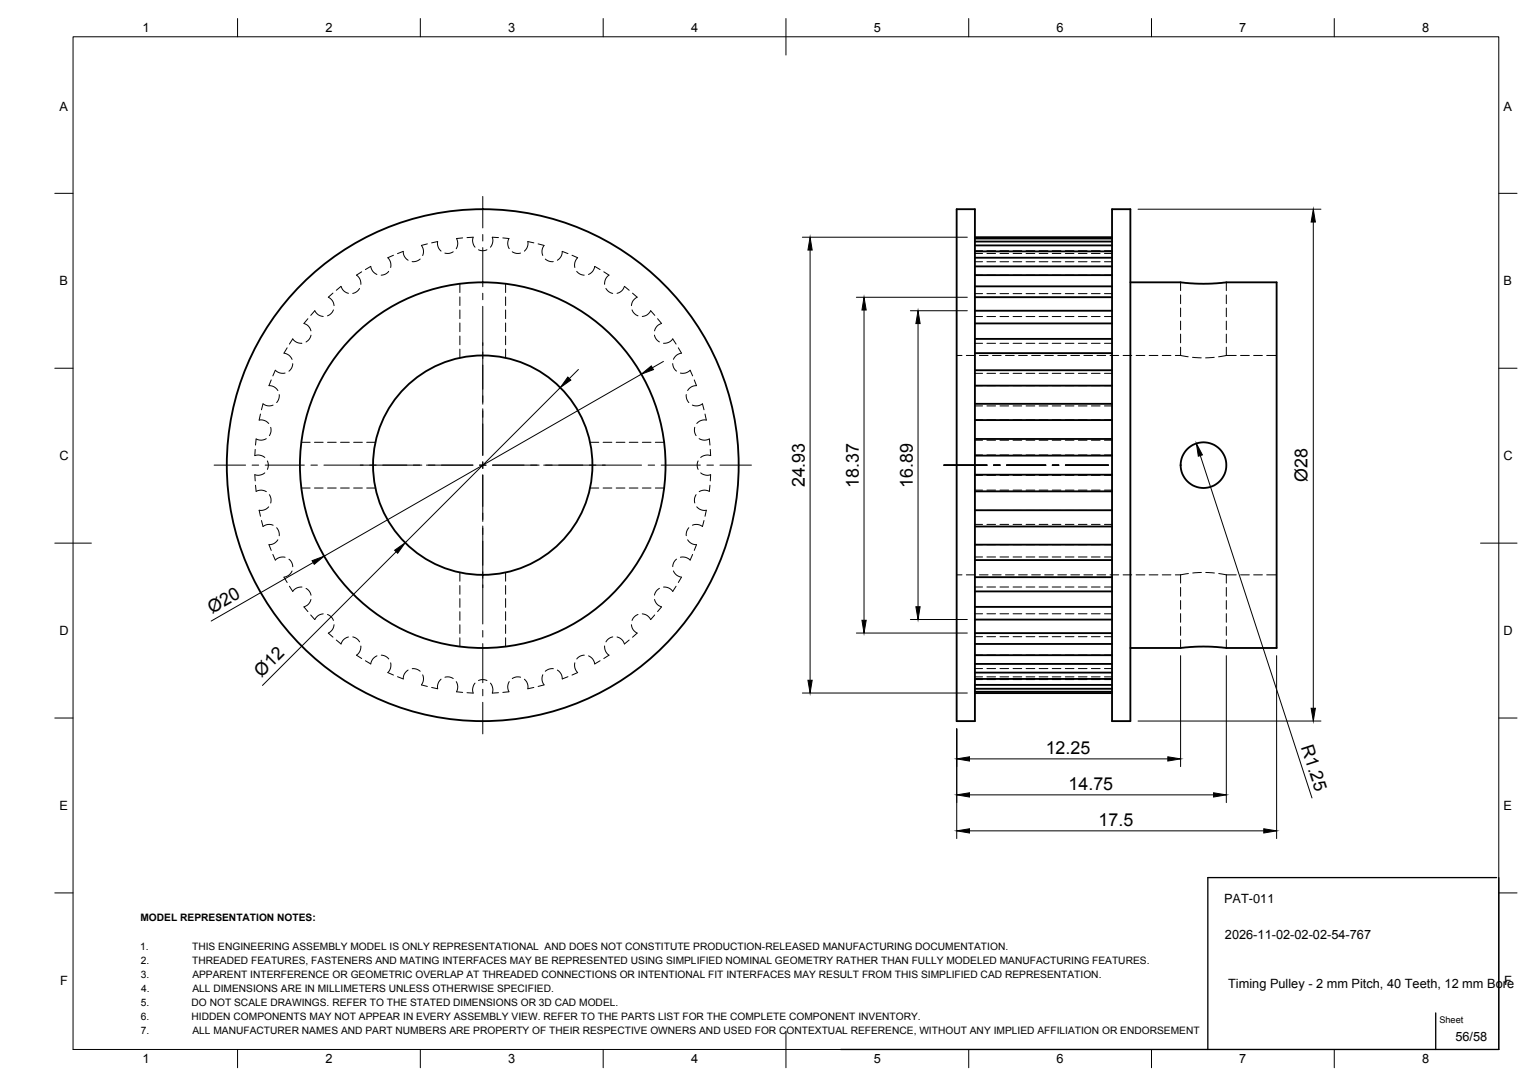
ISO-10303-21;
HEADER;
/* Generated by software containing ST-Developer
 * from STEP Tools, Inc. (www.steptools.com) 
 */

FILE_DESCRIPTION(
/* description */ ('Belt tension measurement rig'),
/* implementation_level */ '2;1');

FILE_NAME(
/* name */ 'Timing Pulley - 2 mm Pitch, 40 Teeth, 12 mm Bore.step',
/* time_stamp */ '2026-10-28T03:24:44-07:00',
/* author */ (''),
/* organization */ (''),
/* preprocessor_version */ 'ST-DEVELOPER v20.2',
/* originating_system */ 'Autodesk Translation Framework v15.17.0.0',
/* authorisation */ '');

FILE_SCHEMA (('AUTOMOTIVE_DESIGN { 1 0 10303 214 3 1 1 }'));
ENDSEC;

DATA;
#10=MECHANICAL_DESIGN_GEOMETRIC_PRESENTATION_REPRESENTATION('',(#757),#23587);
#553=B_SPLINE_CURVE_WITH_KNOTS('',3,(#22249,#22250,#22251,#22252,#22253,
#22254,#22255,#22256,#22257,#22258),.UNSPECIFIED.,.F.,.F.,(4,2,2,2,4),(0.565665723963061,
0.61280433739166,0.659942950820258,0.70708195805217,0.754220965284082),
 .UNSPECIFIED.);
#554=B_SPLINE_CURVE_WITH_KNOTS('',3,(#22260,#22261,#22262,#22263,#22264,
#22265,#22266,#22267,#22268,#22269,#22270,#22271,#22272,#22273,#22274,#22275,
#22276,#22277),.UNSPECIFIED.,.F.,.F.,(4,2,2,2,2,2,2,2,4),(0.18855524132102,
0.235693854749619,0.282832468178217,0.329971475410129,0.377110482642041,
0.424249489873953,0.471388497105864,0.518527110534463,0.565665723963061),
 .UNSPECIFIED.);
#555=B_SPLINE_CURVE_WITH_KNOTS('',3,(#22278,#22279,#22280,#22281,#22282,
#22283,#22284,#22285,#22286,#22287),.UNSPECIFIED.,.F.,.F.,(4,2,2,2,4),(0.754220965284082,
0.801359972515993,0.848498979747905,0.895637593176504,0.942776206605102),
 .UNSPECIFIED.);
#556=B_SPLINE_CURVE_WITH_KNOTS('',3,(#22291,#22292,#22293,#22294,#22295,
#22296,#22297,#22298,#22299,#22300),.UNSPECIFIED.,.F.,.F.,(4,2,2,2,4),(0.188940047579712,
0.236173496177583,0.283406944775455,0.330643519967439,0.377880095159423),
 .UNSPECIFIED.);
#557=B_SPLINE_CURVE_WITH_KNOTS('',3,(#22302,#22303,#22304,#22305,#22306,
#22307,#22308,#22309,#22310,#22311),.UNSPECIFIED.,.F.,.F.,(4,2,2,2,4),(0.,
0.0472365751919841,0.0944731503839682,0.14170659898184,0.188940047579712),
 .UNSPECIFIED.);
#558=B_SPLINE_CURVE_WITH_KNOTS('',3,(#22313,#22314,#22315,#22316,#22317,
#22318,#22319,#22320,#22321,#22322),.UNSPECIFIED.,.F.,.F.,(4,2,2,2,4),(0.566820142739135,
0.614053591337007,0.661287039934879,0.708523615126863,0.755760190318847),
 .UNSPECIFIED.);
#559=B_SPLINE_CURVE_WITH_KNOTS('',3,(#22323,#22324,#22325,#22326,#22327,
#22328,#22329,#22330,#22331,#22332),.UNSPECIFIED.,.F.,.F.,(4,2,2,2,4),(0.377880095159423,
0.425116670351408,0.472353245543392,0.519586694141263,0.566820142739135),
 .UNSPECIFIED.);
#560=B_SPLINE_CURVE_WITH_KNOTS('',3,(#22336,#22337,#22338,#22339,#22340,
#22341,#22342,#22343,#22344,#22345,#22346,#22347,#22348,#22349,#22350,#22351,
#22352,#22353),.UNSPECIFIED.,.F.,.F.,(4,2,2,2,2,2,2,2,4),(0.,0.0472365751919841,
0.0944731503839683,0.14170659898184,0.188940047579712,0.236173496177583,
0.283406944775455,0.330643519967439,0.377880095159423),.UNSPECIFIED.);
#561=B_SPLINE_CURVE_WITH_KNOTS('',3,(#22354,#22355,#22356,#22357,#22358,
#22359,#22360,#22361,#22362,#22363,#22364,#22365,#22366,#22367,#22368,#22369,
#22370,#22371),.UNSPECIFIED.,.F.,.F.,(4,2,2,2,2,2,2,2,4),(0.377880095159423,
0.425116670351408,0.472353245543392,0.519586694141263,0.566820142739135,
0.614053591337007,0.661287039934879,0.708523615126863,0.755760190318847),
 .UNSPECIFIED.);
#562=B_SPLINE_CURVE_WITH_KNOTS('',3,(#22375,#22376,#22377,#22378,#22379,
#22380,#22381,#22382,#22383,#22384),.UNSPECIFIED.,.F.,.F.,(4,2,2,2,4),(0.565665723963061,
0.61280433739166,0.659942950820258,0.70708195805217,0.754220965284082),
 .UNSPECIFIED.);
#563=B_SPLINE_CURVE_WITH_KNOTS('',3,(#22386,#22387,#22388,#22389,#22390,
#22391,#22392,#22393,#22394,#22395,#22396,#22397,#22398,#22399,#22400,#22401,
#22402,#22403),.UNSPECIFIED.,.F.,.F.,(4,2,2,2,2,2,2,2,4),(0.18855524132102,
0.235693854749619,0.282832468178217,0.329971475410129,0.377110482642041,
0.424249489873953,0.471388497105864,0.518527110534463,0.565665723963061),
 .UNSPECIFIED.);
#564=B_SPLINE_CURVE_WITH_KNOTS('',3,(#22404,#22405,#22406,#22407,#22408,
#22409,#22410,#22411,#22412,#22413),.UNSPECIFIED.,.F.,.F.,(4,2,2,2,4),(0.754220965284082,
0.801359972515993,0.848498979747905,0.895637593176504,0.942776206605102),
 .UNSPECIFIED.);
#565=B_SPLINE_CURVE_WITH_KNOTS('',3,(#22423,#22424,#22425,#22426,#22427,
#22428,#22429,#22430,#22431,#22432,#22433,#22434,#22435,#22436,#22437,#22438,
#22439,#22440),.UNSPECIFIED.,.F.,.F.,(4,2,2,2,2,2,2,2,4),(0.18855524132102,
0.235693854749619,0.282832468178217,0.329971475410129,0.377110482642041,
0.424249489873953,0.471388497105864,0.518527110534463,0.565665723963061),
 .UNSPECIFIED.);
#566=B_SPLINE_CURVE_WITH_KNOTS('',3,(#22442,#22443,#22444,#22445,#22446,
#22447,#22448,#22449,#22450,#22451),.UNSPECIFIED.,.F.,.F.,(4,2,2,2,4),(0.565665723963061,
0.61280433739166,0.659942950820258,0.70708195805217,0.754220965284082),
 .UNSPECIFIED.);
#567=B_SPLINE_CURVE_WITH_KNOTS('',3,(#22452,#22453,#22454,#22455,#22456,
#22457,#22458,#22459,#22460,#22461),.UNSPECIFIED.,.F.,.F.,(4,2,2,2,4),(0.754220965284082,
0.801359972515993,0.848498979747905,0.895637593176504,0.942776206605102),
 .UNSPECIFIED.);
#568=B_SPLINE_CURVE_WITH_KNOTS('',3,(#22464,#22465,#22466,#22467,#22468,
#22469,#22470,#22471,#22472,#22473,#22474,#22475,#22476,#22477,#22478,#22479,
#22480,#22481),.UNSPECIFIED.,.F.,.F.,(4,2,2,2,2,2,2,2,4),(0.18855524132102,
0.235693854749619,0.282832468178217,0.329971475410129,0.377110482642041,
0.424249489873953,0.471388497105864,0.518527110534463,0.565665723963061),
 .UNSPECIFIED.);
#569=B_SPLINE_CURVE_WITH_KNOTS('',3,(#22483,#22484,#22485,#22486,#22487,
#22488,#22489,#22490,#22491,#22492),.UNSPECIFIED.,.F.,.F.,(4,2,2,2,4),(0.565665723963061,
0.61280433739166,0.659942950820258,0.70708195805217,0.754220965284082),
 .UNSPECIFIED.);
#570=B_SPLINE_CURVE_WITH_KNOTS('',3,(#22493,#22494,#22495,#22496,#22497,
#22498,#22499,#22500,#22501,#22502),.UNSPECIFIED.,.F.,.F.,(4,2,2,2,4),(0.754220965284082,
0.801359972515993,0.848498979747905,0.895637593176504,0.942776206605102),
 .UNSPECIFIED.);
#571=B_SPLINE_CURVE_WITH_KNOTS('',3,(#22507,#22508,#22509,#22510,#22511,
#22512,#22513,#22514,#22515,#22516,#22517,#22518,#22519,#22520,#22521,#22522,
#22523,#22524),.UNSPECIFIED.,.F.,.F.,(4,2,2,2,2,2,2,2,4),(0.,0.0472365751919841,
0.0944731503839683,0.14170659898184,0.188940047579712,0.236173496177583,
0.283406944775455,0.330643519967439,0.377880095159424),.UNSPECIFIED.);
#572=B_SPLINE_CURVE_WITH_KNOTS('',3,(#22525,#22526,#22527,#22528,#22529,
#22530,#22531,#22532,#22533,#22534,#22535,#22536,#22537,#22538,#22539,#22540,
#22541,#22542),.UNSPECIFIED.,.F.,.F.,(4,2,2,2,2,2,2,2,4),(0.377880095159424,
0.425116670351408,0.472353245543392,0.519586694141263,0.566820142739135,
0.614053591337007,0.661287039934879,0.708523615126863,0.755760190318847),
 .UNSPECIFIED.);
#573=B_SPLINE_CURVE_WITH_KNOTS('',3,(#22546,#22547,#22548,#22549,#22550,
#22551,#22552,#22553,#22554,#22555,#22556,#22557,#22558,#22559,#22560,#22561,
#22562,#22563),.UNSPECIFIED.,.F.,.F.,(4,2,2,2,2,2,2,2,4),(0.,0.0472365751919841,
0.0944731503839683,0.14170659898184,0.188940047579712,0.236173496177583,
0.283406944775455,0.330643519967439,0.377880095159423),.UNSPECIFIED.);
#574=B_SPLINE_CURVE_WITH_KNOTS('',3,(#22564,#22565,#22566,#22567,#22568,
#22569,#22570,#22571,#22572,#22573,#22574,#22575,#22576,#22577,#22578,#22579,
#22580,#22581),.UNSPECIFIED.,.F.,.F.,(4,2,2,2,2,2,2,2,4),(0.377880095159423,
0.425116670351408,0.472353245543392,0.519586694141263,0.566820142739135,
0.614053591337007,0.661287039934879,0.708523615126863,0.755760190318847),
 .UNSPECIFIED.);
#632=SHAPE_REPRESENTATION_RELATIONSHIP('SRR','None',#23883,#687);
#687=ADVANCED_BREP_SHAPE_REPRESENTATION('',(#825),#23581);
#757=STYLED_ITEM('',(#24204),#825);
#825=MANIFOLD_SOLID_BREP('Body1',#12264);
#1015=FACE_BOUND('',#2803,.T.);
#1016=FACE_BOUND('',#2804,.T.);
#1017=FACE_BOUND('',#2805,.T.);
#1018=FACE_BOUND('',#2809,.T.);
#1019=FACE_BOUND('',#2810,.T.);
#1020=FACE_BOUND('',#2811,.T.);
#1021=FACE_BOUND('',#2813,.T.);
#1022=FACE_BOUND('',#2815,.T.);
#1023=FACE_BOUND('',#2818,.T.);
#1024=FACE_BOUND('',#2820,.T.);
#1025=FACE_BOUND('',#2823,.T.);
#1314=PLANE('',#14082);
#1315=PLANE('',#14083);
#1316=PLANE('',#14167);
#1317=PLANE('',#14168);
#1318=PLANE('',#14252);
#1910=FACE_OUTER_BOUND('',#2800,.T.);
#1911=FACE_OUTER_BOUND('',#2801,.T.);
#1912=FACE_OUTER_BOUND('',#2802,.T.);
#1913=FACE_OUTER_BOUND('',#2806,.T.);
#1914=FACE_OUTER_BOUND('',#2807,.T.);
#1915=FACE_OUTER_BOUND('',#2808,.T.);
#1916=FACE_OUTER_BOUND('',#2812,.T.);
#1917=FACE_OUTER_BOUND('',#2814,.T.);
#1918=FACE_OUTER_BOUND('',#2816,.T.);
#1919=FACE_OUTER_BOUND('',#2817,.T.);
#1920=FACE_OUTER_BOUND('',#2819,.T.);
#1921=FACE_OUTER_BOUND('',#2821,.T.);
#1922=FACE_OUTER_BOUND('',#2822,.T.);
#1923=FACE_OUTER_BOUND('',#2824,.T.);
#1924=FACE_OUTER_BOUND('',#2825,.T.);
#1925=FACE_OUTER_BOUND('',#2826,.T.);
#1926=FACE_OUTER_BOUND('',#2827,.T.);
#1927=FACE_OUTER_BOUND('',#2828,.T.);
#1928=FACE_OUTER_BOUND('',#2829,.T.);
#1929=FACE_OUTER_BOUND('',#2830,.T.);
#1930=FACE_OUTER_BOUND('',#2831,.T.);
#1931=FACE_OUTER_BOUND('',#2832,.T.);
#1932=FACE_OUTER_BOUND('',#2833,.T.);
#1933=FACE_OUTER_BOUND('',#2834,.T.);
#1934=FACE_OUTER_BOUND('',#2835,.T.);
#1935=FACE_OUTER_BOUND('',#2836,.T.);
#1936=FACE_OUTER_BOUND('',#2837,.T.);
#1937=FACE_OUTER_BOUND('',#2838,.T.);
#1938=FACE_OUTER_BOUND('',#2839,.T.);
#1939=FACE_OUTER_BOUND('',#2840,.T.);
#1940=FACE_OUTER_BOUND('',#2841,.T.);
#1941=FACE_OUTER_BOUND('',#2842,.T.);
#1942=FACE_OUTER_BOUND('',#2843,.T.);
#1943=FACE_OUTER_BOUND('',#2844,.T.);
#1944=FACE_OUTER_BOUND('',#2845,.T.);
#1945=FACE_OUTER_BOUND('',#2846,.T.);
#1946=FACE_OUTER_BOUND('',#2847,.T.);
#1947=FACE_OUTER_BOUND('',#2848,.T.);
#1948=FACE_OUTER_BOUND('',#2849,.T.);
#1949=FACE_OUTER_BOUND('',#2850,.T.);
#1950=FACE_OUTER_BOUND('',#2851,.T.);
#1951=FACE_OUTER_BOUND('',#2852,.T.);
#1952=FACE_OUTER_BOUND('',#2853,.T.);
#1953=FACE_OUTER_BOUND('',#2854,.T.);
#1954=FACE_OUTER_BOUND('',#2855,.T.);
#1955=FACE_OUTER_BOUND('',#2856,.T.);
#1956=FACE_OUTER_BOUND('',#2857,.T.);
#1957=FACE_OUTER_BOUND('',#2858,.T.);
#1958=FACE_OUTER_BOUND('',#2859,.T.);
#1959=FACE_OUTER_BOUND('',#2860,.T.);
#1960=FACE_OUTER_BOUND('',#2861,.T.);
#1961=FACE_OUTER_BOUND('',#2862,.T.);
#1962=FACE_OUTER_BOUND('',#2863,.T.);
#1963=FACE_OUTER_BOUND('',#2864,.T.);
#1964=FACE_OUTER_BOUND('',#2865,.T.);
#1965=FACE_OUTER_BOUND('',#2866,.T.);
#1966=FACE_OUTER_BOUND('',#2867,.T.);
#1967=FACE_OUTER_BOUND('',#2868,.T.);
#1968=FACE_OUTER_BOUND('',#2869,.T.);
#1969=FACE_OUTER_BOUND('',#2870,.T.);
#1970=FACE_OUTER_BOUND('',#2871,.T.);
#1971=FACE_OUTER_BOUND('',#2872,.T.);
#1972=FACE_OUTER_BOUND('',#2873,.T.);
#1973=FACE_OUTER_BOUND('',#2874,.T.);
#1974=FACE_OUTER_BOUND('',#2875,.T.);
#1975=FACE_OUTER_BOUND('',#2876,.T.);
#1976=FACE_OUTER_BOUND('',#2877,.T.);
#1977=FACE_OUTER_BOUND('',#2878,.T.);
#1978=FACE_OUTER_BOUND('',#2879,.T.);
#1979=FACE_OUTER_BOUND('',#2880,.T.);
#1980=FACE_OUTER_BOUND('',#2881,.T.);
#1981=FACE_OUTER_BOUND('',#2882,.T.);
#1982=FACE_OUTER_BOUND('',#2883,.T.);
#1983=FACE_OUTER_BOUND('',#2884,.T.);
#1984=FACE_OUTER_BOUND('',#2885,.T.);
#1985=FACE_OUTER_BOUND('',#2886,.T.);
#1986=FACE_OUTER_BOUND('',#2887,.T.);
#1987=FACE_OUTER_BOUND('',#2888,.T.);
#1988=FACE_OUTER_BOUND('',#2889,.T.);
#1989=FACE_OUTER_BOUND('',#2890,.T.);
#1990=FACE_OUTER_BOUND('',#2891,.T.);
#1991=FACE_OUTER_BOUND('',#2892,.T.);
#1992=FACE_OUTER_BOUND('',#2893,.T.);
#1993=FACE_OUTER_BOUND('',#2894,.T.);
#1994=FACE_OUTER_BOUND('',#2895,.T.);
#1995=FACE_OUTER_BOUND('',#2896,.T.);
#1996=FACE_OUTER_BOUND('',#2897,.T.);
#1997=FACE_OUTER_BOUND('',#2898,.T.);
#1998=FACE_OUTER_BOUND('',#2899,.T.);
#1999=FACE_OUTER_BOUND('',#2900,.T.);
#2000=FACE_OUTER_BOUND('',#2901,.T.);
#2001=FACE_OUTER_BOUND('',#2902,.T.);
#2002=FACE_OUTER_BOUND('',#2903,.T.);
#2800=EDGE_LOOP('',(#10396,#10397,#10398,#10399,#10400,#10401,#10402,#10403,
#10404));
#2801=EDGE_LOOP('',(#10405,#10406,#10407,#10408,#10409,#10410,#10411));
#2802=EDGE_LOOP('',(#10412,#10413,#10414,#10415,#10416,#10417,#10418,#10419,
#10420));
#2803=EDGE_LOOP('',(#10421,#10422,#10423));
#2804=EDGE_LOOP('',(#10424,#10425,#10426));
#2805=EDGE_LOOP('',(#10427,#10428,#10429));
#2806=EDGE_LOOP('',(#10430,#10431,#10432,#10433,#10434,#10435,#10436));
#2807=EDGE_LOOP('',(#10437,#10438,#10439,#10440,#10441,#10442,#10443));
#2808=EDGE_LOOP('',(#10444,#10445,#10446,#10447,#10448,#10449,#10450,#10451,
#10452,#10453));
#2809=EDGE_LOOP('',(#10454,#10455));
#2810=EDGE_LOOP('',(#10456,#10457));
#2811=EDGE_LOOP('',(#10458,#10459));
#2812=EDGE_LOOP('',(#10460));
#2813=EDGE_LOOP('',(#10461));
#2814=EDGE_LOOP('',(#10462));
#2815=EDGE_LOOP('',(#10463,#10464,#10465,#10466,#10467,#10468,#10469,#10470,
#10471,#10472,#10473,#10474,#10475,#10476,#10477,#10478,#10479,#10480,#10481,
#10482,#10483,#10484,#10485,#10486,#10487,#10488,#10489,#10490,#10491,#10492,
#10493,#10494,#10495,#10496,#10497,#10498,#10499,#10500,#10501,#10502,#10503,
#10504,#10505,#10506,#10507,#10508,#10509,#10510,#10511,#10512,#10513,#10514,
#10515,#10516,#10517,#10518,#10519,#10520,#10521,#10522,#10523,#10524,#10525,
#10526,#10527,#10528,#10529,#10530,#10531,#10532,#10533,#10534,#10535,#10536,
#10537,#10538,#10539,#10540,#10541,#10542));
#2816=EDGE_LOOP('',(#10543,#10544,#10545,#10546));
#2817=EDGE_LOOP('',(#10547));
#2818=EDGE_LOOP('',(#10548));
#2819=EDGE_LOOP('',(#10549));
#2820=EDGE_LOOP('',(#10550,#10551,#10552,#10553,#10554,#10555,#10556,#10557,
#10558,#10559,#10560,#10561,#10562,#10563,#10564,#10565,#10566,#10567,#10568,
#10569,#10570,#10571,#10572,#10573,#10574,#10575,#10576,#10577,#10578,#10579,
#10580,#10581,#10582,#10583,#10584,#10585,#10586,#10587,#10588,#10589,#10590,
#10591,#10592,#10593,#10594,#10595,#10596,#10597,#10598,#10599,#10600,#10601,
#10602,#10603,#10604,#10605,#10606,#10607,#10608,#10609,#10610,#10611,#10612,
#10613,#10614,#10615,#10616,#10617,#10618,#10619,#10620,#10621,#10622,#10623,
#10624,#10625,#10626,#10627,#10628,#10629));
#2821=EDGE_LOOP('',(#10630,#10631,#10632,#10633));
#2822=EDGE_LOOP('',(#10634));
#2823=EDGE_LOOP('',(#10635));
#2824=EDGE_LOOP('',(#10636,#10637,#10638,#10639));
#2825=EDGE_LOOP('',(#10640,#10641,#10642,#10643));
#2826=EDGE_LOOP('',(#10644,#10645,#10646,#10647));
#2827=EDGE_LOOP('',(#10648,#10649,#10650,#10651));
#2828=EDGE_LOOP('',(#10652,#10653,#10654,#10655));
#2829=EDGE_LOOP('',(#10656,#10657,#10658,#10659));
#2830=EDGE_LOOP('',(#10660,#10661,#10662,#10663));
#2831=EDGE_LOOP('',(#10664,#10665,#10666,#10667));
#2832=EDGE_LOOP('',(#10668,#10669,#10670,#10671));
#2833=EDGE_LOOP('',(#10672,#10673,#10674,#10675));
#2834=EDGE_LOOP('',(#10676,#10677,#10678,#10679));
#2835=EDGE_LOOP('',(#10680,#10681,#10682,#10683));
#2836=EDGE_LOOP('',(#10684,#10685,#10686,#10687));
#2837=EDGE_LOOP('',(#10688,#10689,#10690,#10691));
#2838=EDGE_LOOP('',(#10692,#10693,#10694,#10695));
#2839=EDGE_LOOP('',(#10696,#10697,#10698,#10699));
#2840=EDGE_LOOP('',(#10700,#10701,#10702,#10703));
#2841=EDGE_LOOP('',(#10704,#10705,#10706,#10707));
#2842=EDGE_LOOP('',(#10708,#10709,#10710,#10711));
#2843=EDGE_LOOP('',(#10712,#10713,#10714,#10715));
#2844=EDGE_LOOP('',(#10716,#10717,#10718,#10719));
#2845=EDGE_LOOP('',(#10720,#10721,#10722,#10723));
#2846=EDGE_LOOP('',(#10724,#10725,#10726,#10727));
#2847=EDGE_LOOP('',(#10728,#10729,#10730,#10731));
#2848=EDGE_LOOP('',(#10732,#10733,#10734,#10735));
#2849=EDGE_LOOP('',(#10736,#10737,#10738,#10739));
#2850=EDGE_LOOP('',(#10740,#10741,#10742,#10743));
#2851=EDGE_LOOP('',(#10744,#10745,#10746,#10747));
#2852=EDGE_LOOP('',(#10748,#10749,#10750,#10751));
#2853=EDGE_LOOP('',(#10752,#10753,#10754,#10755));
#2854=EDGE_LOOP('',(#10756,#10757,#10758,#10759));
#2855=EDGE_LOOP('',(#10760,#10761,#10762,#10763));
#2856=EDGE_LOOP('',(#10764,#10765,#10766,#10767));
#2857=EDGE_LOOP('',(#10768,#10769,#10770,#10771));
#2858=EDGE_LOOP('',(#10772,#10773,#10774,#10775));
#2859=EDGE_LOOP('',(#10776,#10777,#10778,#10779));
#2860=EDGE_LOOP('',(#10780,#10781,#10782,#10783));
#2861=EDGE_LOOP('',(#10784,#10785,#10786,#10787));
#2862=EDGE_LOOP('',(#10788,#10789,#10790,#10791));
#2863=EDGE_LOOP('',(#10792,#10793,#10794,#10795));
#2864=EDGE_LOOP('',(#10796,#10797,#10798,#10799));
#2865=EDGE_LOOP('',(#10800,#10801,#10802,#10803));
#2866=EDGE_LOOP('',(#10804,#10805,#10806,#10807));
#2867=EDGE_LOOP('',(#10808,#10809,#10810,#10811));
#2868=EDGE_LOOP('',(#10812,#10813,#10814,#10815));
#2869=EDGE_LOOP('',(#10816,#10817,#10818,#10819));
#2870=EDGE_LOOP('',(#10820,#10821,#10822,#10823));
#2871=EDGE_LOOP('',(#10824,#10825,#10826,#10827));
#2872=EDGE_LOOP('',(#10828,#10829,#10830,#10831));
#2873=EDGE_LOOP('',(#10832,#10833,#10834,#10835));
#2874=EDGE_LOOP('',(#10836,#10837,#10838,#10839));
#2875=EDGE_LOOP('',(#10840,#10841,#10842,#10843));
#2876=EDGE_LOOP('',(#10844,#10845,#10846,#10847));
#2877=EDGE_LOOP('',(#10848,#10849,#10850,#10851));
#2878=EDGE_LOOP('',(#10852,#10853,#10854,#10855));
#2879=EDGE_LOOP('',(#10856,#10857,#10858,#10859));
#2880=EDGE_LOOP('',(#10860,#10861,#10862,#10863));
#2881=EDGE_LOOP('',(#10864,#10865,#10866,#10867));
#2882=EDGE_LOOP('',(#10868,#10869,#10870,#10871));
#2883=EDGE_LOOP('',(#10872,#10873,#10874,#10875));
#2884=EDGE_LOOP('',(#10876,#10877,#10878,#10879));
#2885=EDGE_LOOP('',(#10880,#10881,#10882,#10883));
#2886=EDGE_LOOP('',(#10884,#10885,#10886,#10887));
#2887=EDGE_LOOP('',(#10888,#10889,#10890,#10891));
#2888=EDGE_LOOP('',(#10892,#10893,#10894,#10895));
#2889=EDGE_LOOP('',(#10896,#10897,#10898,#10899));
#2890=EDGE_LOOP('',(#10900,#10901,#10902,#10903));
#2891=EDGE_LOOP('',(#10904,#10905,#10906,#10907));
#2892=EDGE_LOOP('',(#10908,#10909,#10910,#10911));
#2893=EDGE_LOOP('',(#10912,#10913,#10914,#10915));
#2894=EDGE_LOOP('',(#10916,#10917,#10918,#10919));
#2895=EDGE_LOOP('',(#10920,#10921,#10922,#10923));
#2896=EDGE_LOOP('',(#10924,#10925,#10926,#10927));
#2897=EDGE_LOOP('',(#10928,#10929,#10930,#10931));
#2898=EDGE_LOOP('',(#10932,#10933,#10934,#10935));
#2899=EDGE_LOOP('',(#10936,#10937,#10938,#10939));
#2900=EDGE_LOOP('',(#10940,#10941,#10942,#10943));
#2901=EDGE_LOOP('',(#10944,#10945,#10946,#10947));
#2902=EDGE_LOOP('',(#10948,#10949,#10950,#10951));
#2903=EDGE_LOOP('',(#10952,#10953,#10954,#10955));
#3569=LINE('',#22289,#4320);
#3570=LINE('',#22373,#4321);
#3571=LINE('',#22417,#4322);
#3572=LINE('',#22419,#4323);
#3573=LINE('',#22505,#4324);
#3574=LINE('',#22582,#4325);
#3575=LINE('',#22586,#4326);
#3576=LINE('',#22588,#4327);
#3577=LINE('',#22757,#4328);
#3578=LINE('',#22925,#4329);
#3579=LINE('',#22928,#4330);
#3580=LINE('',#22929,#4331);
#3581=LINE('',#22931,#4332);
#3582=LINE('',#22933,#4333);
#3583=LINE('',#22935,#4334);
#3584=LINE('',#22937,#4335);
#3585=LINE('',#22939,#4336);
#3586=LINE('',#22941,#4337);
#3587=LINE('',#22943,#4338);
#3588=LINE('',#22945,#4339);
#3589=LINE('',#22947,#4340);
#3590=LINE('',#22949,#4341);
#3591=LINE('',#22951,#4342);
#3592=LINE('',#22953,#4343);
#3593=LINE('',#22955,#4344);
#3594=LINE('',#22957,#4345);
#3595=LINE('',#22959,#4346);
#3596=LINE('',#22961,#4347);
#3597=LINE('',#22963,#4348);
#3598=LINE('',#22965,#4349);
#3599=LINE('',#22967,#4350);
#3600=LINE('',#22969,#4351);
#3601=LINE('',#22971,#4352);
#3602=LINE('',#22973,#4353);
#3603=LINE('',#22975,#4354);
#3604=LINE('',#22977,#4355);
#3605=LINE('',#22979,#4356);
#3606=LINE('',#22981,#4357);
#3607=LINE('',#22983,#4358);
#3608=LINE('',#22985,#4359);
#3609=LINE('',#22987,#4360);
#3610=LINE('',#22989,#4361);
#3611=LINE('',#22991,#4362);
#3612=LINE('',#22993,#4363);
#3613=LINE('',#22995,#4364);
#3614=LINE('',#22997,#4365);
#3615=LINE('',#22999,#4366);
#3616=LINE('',#23001,#4367);
#3617=LINE('',#23003,#4368);
#3618=LINE('',#23005,#4369);
#3619=LINE('',#23007,#4370);
#3620=LINE('',#23009,#4371);
#3621=LINE('',#23011,#4372);
#3622=LINE('',#23013,#4373);
#3623=LINE('',#23015,#4374);
#3624=LINE('',#23017,#4375);
#3625=LINE('',#23019,#4376);
#3626=LINE('',#23021,#4377);
#3627=LINE('',#23023,#4378);
#3628=LINE('',#23025,#4379);
#3629=LINE('',#23027,#4380);
#3630=LINE('',#23029,#4381);
#3631=LINE('',#23031,#4382);
#3632=LINE('',#23033,#4383);
#3633=LINE('',#23035,#4384);
#3634=LINE('',#23037,#4385);
#3635=LINE('',#23039,#4386);
#3636=LINE('',#23041,#4387);
#3637=LINE('',#23043,#4388);
#3638=LINE('',#23045,#4389);
#3639=LINE('',#23047,#4390);
#3640=LINE('',#23049,#4391);
#3641=LINE('',#23051,#4392);
#3642=LINE('',#23053,#4393);
#3643=LINE('',#23055,#4394);
#3644=LINE('',#23057,#4395);
#3645=LINE('',#23059,#4396);
#3646=LINE('',#23061,#4397);
#3647=LINE('',#23063,#4398);
#3648=LINE('',#23065,#4399);
#3649=LINE('',#23067,#4400);
#3650=LINE('',#23069,#4401);
#3651=LINE('',#23071,#4402);
#3652=LINE('',#23073,#4403);
#3653=LINE('',#23075,#4404);
#3654=LINE('',#23077,#4405);
#3655=LINE('',#23079,#4406);
#3656=LINE('',#23081,#4407);
#3657=LINE('',#23083,#4408);
#3658=LINE('',#23085,#4409);
#4320=VECTOR('',#17512,0.125);
#4321=VECTOR('',#17515,0.125);
#4322=VECTOR('',#17520,1.);
#4323=VECTOR('',#17521,1.);
#4324=VECTOR('',#17526,0.125);
#4325=VECTOR('',#17529,0.125);
#4326=VECTOR('',#17534,0.6);
#4327=VECTOR('',#17535,0.6);
#4328=VECTOR('',#17708,1.4);
#4329=VECTOR('',#17879,1.4);
#4330=VECTOR('',#17884,1.);
#4331=VECTOR('',#17885,1.);
#4332=VECTOR('',#17888,1.);
#4333=VECTOR('',#17891,1.);
#4334=VECTOR('',#17894,1.);
#4335=VECTOR('',#17897,1.);
#4336=VECTOR('',#17900,1.);
#4337=VECTOR('',#17903,1.);
#4338=VECTOR('',#17906,1.);
#4339=VECTOR('',#17909,1.);
#4340=VECTOR('',#17912,1.);
#4341=VECTOR('',#17915,1.);
#4342=VECTOR('',#17918,1.);
#4343=VECTOR('',#17921,1.);
#4344=VECTOR('',#17924,1.);
#4345=VECTOR('',#17927,1.);
#4346=VECTOR('',#17930,1.);
#4347=VECTOR('',#17933,1.);
#4348=VECTOR('',#17936,1.);
#4349=VECTOR('',#17939,1.);
#4350=VECTOR('',#17942,1.);
#4351=VECTOR('',#17945,1.);
#4352=VECTOR('',#17948,1.);
#4353=VECTOR('',#17951,1.);
#4354=VECTOR('',#17954,1.);
#4355=VECTOR('',#17957,1.);
#4356=VECTOR('',#17960,1.);
#4357=VECTOR('',#17963,1.);
#4358=VECTOR('',#17966,1.);
#4359=VECTOR('',#17969,1.);
#4360=VECTOR('',#17972,1.);
#4361=VECTOR('',#17975,1.);
#4362=VECTOR('',#17978,1.);
#4363=VECTOR('',#17981,1.);
#4364=VECTOR('',#17984,1.);
#4365=VECTOR('',#17987,1.);
#4366=VECTOR('',#17990,1.);
#4367=VECTOR('',#17993,1.);
#4368=VECTOR('',#17996,1.);
#4369=VECTOR('',#17999,1.);
#4370=VECTOR('',#18002,1.);
#4371=VECTOR('',#18005,1.);
#4372=VECTOR('',#18008,1.);
#4373=VECTOR('',#18011,1.);
#4374=VECTOR('',#18014,1.);
#4375=VECTOR('',#18017,1.);
#4376=VECTOR('',#18020,1.);
#4377=VECTOR('',#18023,1.);
#4378=VECTOR('',#18026,1.);
#4379=VECTOR('',#18029,1.);
#4380=VECTOR('',#18032,1.);
#4381=VECTOR('',#18035,1.);
#4382=VECTOR('',#18038,1.);
#4383=VECTOR('',#18041,1.);
#4384=VECTOR('',#18044,1.);
#4385=VECTOR('',#18047,1.);
#4386=VECTOR('',#18050,1.);
#4387=VECTOR('',#18053,1.);
#4388=VECTOR('',#18056,1.);
#4389=VECTOR('',#18059,1.);
#4390=VECTOR('',#18062,1.);
#4391=VECTOR('',#18065,1.);
#4392=VECTOR('',#18068,1.);
#4393=VECTOR('',#18071,1.);
#4394=VECTOR('',#18074,1.);
#4395=VECTOR('',#18077,1.);
#4396=VECTOR('',#18080,1.);
#4397=VECTOR('',#18083,1.);
#4398=VECTOR('',#18086,1.);
#4399=VECTOR('',#18089,1.);
#4400=VECTOR('',#18092,1.);
#4401=VECTOR('',#18095,1.);
#4402=VECTOR('',#18098,1.);
#4403=VECTOR('',#18101,1.);
#4404=VECTOR('',#18104,1.);
#4405=VECTOR('',#18107,1.);
#4406=VECTOR('',#18110,1.);
#4407=VECTOR('',#18113,1.);
#4408=VECTOR('',#18116,1.);
#4409=VECTOR('',#18119,1.);
#5036=CIRCLE('',#14075,1.);
#5037=CIRCLE('',#14076,1.);
#5038=CIRCLE('',#14080,0.6);
#5039=CIRCLE('',#14081,0.6);
#5040=CIRCLE('',#14084,1.4);
#5041=CIRCLE('',#14085,0.0555000000000001);
#5042=CIRCLE('',#14086,1.24783954473516);
#5043=CIRCLE('',#14087,0.0555000000000001);
#5044=CIRCLE('',#14088,1.24783954473516);
#5045=CIRCLE('',#14089,0.0555000000000001);
#5046=CIRCLE('',#14090,1.24783954473516);
#5047=CIRCLE('',#14091,0.0555000000000001);
#5048=CIRCLE('',#14092,1.24783954473516);
#5049=CIRCLE('',#14093,0.0555000000000001);
#5050=CIRCLE('',#14094,1.24783954473516);
#5051=CIRCLE('',#14095,0.0555000000000001);
#5052=CIRCLE('',#14096,1.24783954473516);
#5053=CIRCLE('',#14097,0.0555000000000001);
#5054=CIRCLE('',#14098,1.24783954473516);
#5055=CIRCLE('',#14099,0.0555000000000001);
#5056=CIRCLE('',#14100,1.24783954473516);
#5057=CIRCLE('',#14101,0.0555000000000001);
#5058=CIRCLE('',#14102,1.24783954473516);
#5059=CIRCLE('',#14103,0.0555000000000001);
#5060=CIRCLE('',#14104,1.24783954473516);
#5061=CIRCLE('',#14105,0.0555000000000001);
#5062=CIRCLE('',#14106,1.24783954473516);
#5063=CIRCLE('',#14107,0.0555000000000001);
#5064=CIRCLE('',#14108,1.24783954473516);
#5065=CIRCLE('',#14109,0.0555000000000001);
#5066=CIRCLE('',#14110,1.24783954473516);
#5067=CIRCLE('',#14111,0.0555000000000001);
#5068=CIRCLE('',#14112,1.24783954473516);
#5069=CIRCLE('',#14113,0.0555000000000001);
#5070=CIRCLE('',#14114,1.24783954473516);
#5071=CIRCLE('',#14115,0.0555000000000001);
#5072=CIRCLE('',#14116,1.24783954473516);
#5073=CIRCLE('',#14117,0.0555000000000001);
#5074=CIRCLE('',#14118,1.24783954473516);
#5075=CIRCLE('',#14119,0.0555000000000001);
#5076=CIRCLE('',#14120,1.24783954473516);
#5077=CIRCLE('',#14121,0.0555000000000001);
#5078=CIRCLE('',#14122,1.24783954473516);
#5079=CIRCLE('',#14123,0.0555000000000001);
#5080=CIRCLE('',#14124,1.24783954473516);
#5081=CIRCLE('',#14125,0.0555000000000001);
#5082=CIRCLE('',#14126,1.24783954473516);
#5083=CIRCLE('',#14127,0.0555000000000001);
#5084=CIRCLE('',#14128,1.24783954473516);
#5085=CIRCLE('',#14129,0.0555000000000001);
#5086=CIRCLE('',#14130,1.24783954473516);
#5087=CIRCLE('',#14131,0.0555000000000001);
#5088=CIRCLE('',#14132,1.24783954473516);
#5089=CIRCLE('',#14133,0.0555000000000001);
#5090=CIRCLE('',#14134,1.24783954473516);
#5091=CIRCLE('',#14135,0.0555000000000001);
#5092=CIRCLE('',#14136,1.24783954473516);
#5093=CIRCLE('',#14137,0.0555000000000001);
#5094=CIRCLE('',#14138,1.24783954473516);
#5095=CIRCLE('',#14139,0.0555000000000001);
#5096=CIRCLE('',#14140,1.24783954473516);
#5097=CIRCLE('',#14141,0.0555000000000001);
#5098=CIRCLE('',#14142,1.24783954473516);
#5099=CIRCLE('',#14143,0.0555000000000001);
#5100=CIRCLE('',#14144,1.24783954473516);
#5101=CIRCLE('',#14145,0.0555000000000001);
#5102=CIRCLE('',#14146,1.24783954473516);
#5103=CIRCLE('',#14147,0.0555000000000001);
#5104=CIRCLE('',#14148,1.24783954473516);
#5105=CIRCLE('',#14149,0.0555000000000001);
#5106=CIRCLE('',#14150,1.24783954473516);
#5107=CIRCLE('',#14151,0.0555000000000001);
#5108=CIRCLE('',#14152,1.24783954473516);
#5109=CIRCLE('',#14153,0.0555000000000001);
#5110=CIRCLE('',#14154,1.24783954473516);
#5111=CIRCLE('',#14155,0.0555000000000001);
#5112=CIRCLE('',#14156,1.24783954473516);
#5113=CIRCLE('',#14157,0.0555000000000001);
#5114=CIRCLE('',#14158,1.24783954473516);
#5115=CIRCLE('',#14159,0.0555000000000001);
#5116=CIRCLE('',#14160,1.24783954473516);
#5117=CIRCLE('',#14161,0.0555000000000001);
#5118=CIRCLE('',#14162,1.24783954473516);
#5119=CIRCLE('',#14163,0.0555000000000001);
#5120=CIRCLE('',#14164,1.24783954473516);
#5121=CIRCLE('',#14166,1.4);
#5122=CIRCLE('',#14169,1.4);
#5123=CIRCLE('',#14170,0.0555000000000001);
#5124=CIRCLE('',#14171,1.24783954473516);
#5125=CIRCLE('',#14172,0.0555000000000001);
#5126=CIRCLE('',#14173,1.24783954473516);
#5127=CIRCLE('',#14174,0.0555000000000001);
#5128=CIRCLE('',#14175,1.24783954473516);
#5129=CIRCLE('',#14176,0.0555000000000001);
#5130=CIRCLE('',#14177,1.24783954473516);
#5131=CIRCLE('',#14178,0.0555000000000001);
#5132=CIRCLE('',#14179,1.24783954473516);
#5133=CIRCLE('',#14180,0.0555000000000001);
#5134=CIRCLE('',#14181,1.24783954473516);
#5135=CIRCLE('',#14182,0.0555000000000001);
#5136=CIRCLE('',#14183,1.24783954473516);
#5137=CIRCLE('',#14184,0.0555000000000001);
#5138=CIRCLE('',#14185,1.24783954473516);
#5139=CIRCLE('',#14186,0.0555000000000001);
#5140=CIRCLE('',#14187,1.24783954473516);
#5141=CIRCLE('',#14188,0.0555000000000001);
#5142=CIRCLE('',#14189,1.24783954473516);
#5143=CIRCLE('',#14190,0.0555000000000001);
#5144=CIRCLE('',#14191,1.24783954473516);
#5145=CIRCLE('',#14192,0.0555000000000001);
#5146=CIRCLE('',#14193,1.24783954473516);
#5147=CIRCLE('',#14194,0.0555000000000001);
#5148=CIRCLE('',#14195,1.24783954473516);
#5149=CIRCLE('',#14196,0.0555000000000001);
#5150=CIRCLE('',#14197,1.24783954473516);
#5151=CIRCLE('',#14198,0.0555000000000001);
#5152=CIRCLE('',#14199,1.24783954473516);
#5153=CIRCLE('',#14200,0.0555000000000001);
#5154=CIRCLE('',#14201,1.24783954473516);
#5155=CIRCLE('',#14202,0.0555000000000001);
#5156=CIRCLE('',#14203,1.24783954473516);
#5157=CIRCLE('',#14204,0.0555000000000001);
#5158=CIRCLE('',#14205,1.24783954473516);
#5159=CIRCLE('',#14206,0.0555000000000001);
#5160=CIRCLE('',#14207,1.24783954473516);
#5161=CIRCLE('',#14208,0.0555000000000001);
#5162=CIRCLE('',#14209,1.24783954473516);
#5163=CIRCLE('',#14210,0.0555000000000001);
#5164=CIRCLE('',#14211,1.24783954473516);
#5165=CIRCLE('',#14212,0.0555000000000001);
#5166=CIRCLE('',#14213,1.24783954473516);
#5167=CIRCLE('',#14214,0.0555000000000001);
#5168=CIRCLE('',#14215,1.24783954473516);
#5169=CIRCLE('',#14216,0.0555000000000001);
#5170=CIRCLE('',#14217,1.24783954473516);
#5171=CIRCLE('',#14218,0.0555000000000001);
#5172=CIRCLE('',#14219,1.24783954473516);
#5173=CIRCLE('',#14220,0.0555000000000001);
#5174=CIRCLE('',#14221,1.24783954473516);
#5175=CIRCLE('',#14222,0.0555000000000001);
#5176=CIRCLE('',#14223,1.24783954473516);
#5177=CIRCLE('',#14224,0.0555000000000001);
#5178=CIRCLE('',#14225,1.24783954473516);
#5179=CIRCLE('',#14226,0.0555000000000001);
#5180=CIRCLE('',#14227,1.24783954473516);
#5181=CIRCLE('',#14228,0.0555000000000001);
#5182=CIRCLE('',#14229,1.24783954473516);
#5183=CIRCLE('',#14230,0.0555000000000001);
#5184=CIRCLE('',#14231,1.24783954473516);
#5185=CIRCLE('',#14232,0.0555000000000001);
#5186=CIRCLE('',#14233,1.24783954473516);
#5187=CIRCLE('',#14234,0.0555000000000001);
#5188=CIRCLE('',#14235,1.24783954473516);
#5189=CIRCLE('',#14236,0.0555000000000001);
#5190=CIRCLE('',#14237,1.24783954473516);
#5191=CIRCLE('',#14238,0.0555000000000001);
#5192=CIRCLE('',#14239,1.24783954473516);
#5193=CIRCLE('',#14240,0.0555000000000001);
#5194=CIRCLE('',#14241,1.24783954473516);
#5195=CIRCLE('',#14242,0.0555000000000001);
#5196=CIRCLE('',#14243,1.24783954473516);
#5197=CIRCLE('',#14244,0.0555000000000001);
#5198=CIRCLE('',#14245,1.24783954473516);
#5199=CIRCLE('',#14246,0.0555000000000001);
#5200=CIRCLE('',#14247,1.24783954473516);
#5201=CIRCLE('',#14248,0.0555000000000001);
#5202=CIRCLE('',#14249,1.24783954473516);
#5203=CIRCLE('',#14251,1.4);
#6073=VERTEX_POINT('',#22247);
#6074=VERTEX_POINT('',#22248);
#6075=VERTEX_POINT('',#22259);
#6076=VERTEX_POINT('',#22288);
#6077=VERTEX_POINT('',#22290);
#6078=VERTEX_POINT('',#22301);
#6079=VERTEX_POINT('',#22312);
#6080=VERTEX_POINT('',#22334);
#6081=VERTEX_POINT('',#22335);
#6082=VERTEX_POINT('',#22372);
#6083=VERTEX_POINT('',#22374);
#6084=VERTEX_POINT('',#22385);
#6085=VERTEX_POINT('',#22415);
#6086=VERTEX_POINT('',#22418);
#6087=VERTEX_POINT('',#22421);
#6088=VERTEX_POINT('',#22422);
#6089=VERTEX_POINT('',#22441);
#6090=VERTEX_POINT('',#22462);
#6091=VERTEX_POINT('',#22463);
#6092=VERTEX_POINT('',#22482);
#6093=VERTEX_POINT('',#22504);
#6094=VERTEX_POINT('',#22506);
#6095=VERTEX_POINT('',#22544);
#6096=VERTEX_POINT('',#22545);
#6097=VERTEX_POINT('',#22584);
#6098=VERTEX_POINT('',#22587);
#6099=VERTEX_POINT('',#22592);
#6100=VERTEX_POINT('',#22594);
#6101=VERTEX_POINT('',#22595);
#6102=VERTEX_POINT('',#22597);
#6103=VERTEX_POINT('',#22599);
#6104=VERTEX_POINT('',#22601);
#6105=VERTEX_POINT('',#22603);
#6106=VERTEX_POINT('',#22605);
#6107=VERTEX_POINT('',#22607);
#6108=VERTEX_POINT('',#22609);
#6109=VERTEX_POINT('',#22611);
#6110=VERTEX_POINT('',#22613);
#6111=VERTEX_POINT('',#22615);
#6112=VERTEX_POINT('',#22617);
#6113=VERTEX_POINT('',#22619);
#6114=VERTEX_POINT('',#22621);
#6115=VERTEX_POINT('',#22623);
#6116=VERTEX_POINT('',#22625);
#6117=VERTEX_POINT('',#22627);
#6118=VERTEX_POINT('',#22629);
#6119=VERTEX_POINT('',#22631);
#6120=VERTEX_POINT('',#22633);
#6121=VERTEX_POINT('',#22635);
#6122=VERTEX_POINT('',#22637);
#6123=VERTEX_POINT('',#22639);
#6124=VERTEX_POINT('',#22641);
#6125=VERTEX_POINT('',#22643);
#6126=VERTEX_POINT('',#22645);
#6127=VERTEX_POINT('',#22647);
#6128=VERTEX_POINT('',#22649);
#6129=VERTEX_POINT('',#22651);
#6130=VERTEX_POINT('',#22653);
#6131=VERTEX_POINT('',#22655);
#6132=VERTEX_POINT('',#22657);
#6133=VERTEX_POINT('',#22659);
#6134=VERTEX_POINT('',#22661);
#6135=VERTEX_POINT('',#22663);
#6136=VERTEX_POINT('',#22665);
#6137=VERTEX_POINT('',#22667);
#6138=VERTEX_POINT('',#22669);
#6139=VERTEX_POINT('',#22671);
#6140=VERTEX_POINT('',#22673);
#6141=VERTEX_POINT('',#22675);
#6142=VERTEX_POINT('',#22677);
#6143=VERTEX_POINT('',#22679);
#6144=VERTEX_POINT('',#22681);
#6145=VERTEX_POINT('',#22683);
#6146=VERTEX_POINT('',#22685);
#6147=VERTEX_POINT('',#22687);
#6148=VERTEX_POINT('',#22689);
#6149=VERTEX_POINT('',#22691);
#6150=VERTEX_POINT('',#22693);
#6151=VERTEX_POINT('',#22695);
#6152=VERTEX_POINT('',#22697);
#6153=VERTEX_POINT('',#22699);
#6154=VERTEX_POINT('',#22701);
#6155=VERTEX_POINT('',#22703);
#6156=VERTEX_POINT('',#22705);
#6157=VERTEX_POINT('',#22707);
#6158=VERTEX_POINT('',#22709);
#6159=VERTEX_POINT('',#22711);
#6160=VERTEX_POINT('',#22713);
#6161=VERTEX_POINT('',#22715);
#6162=VERTEX_POINT('',#22717);
#6163=VERTEX_POINT('',#22719);
#6164=VERTEX_POINT('',#22721);
#6165=VERTEX_POINT('',#22723);
#6166=VERTEX_POINT('',#22725);
#6167=VERTEX_POINT('',#22727);
#6168=VERTEX_POINT('',#22729);
#6169=VERTEX_POINT('',#22731);
#6170=VERTEX_POINT('',#22733);
#6171=VERTEX_POINT('',#22735);
#6172=VERTEX_POINT('',#22737);
#6173=VERTEX_POINT('',#22739);
#6174=VERTEX_POINT('',#22741);
#6175=VERTEX_POINT('',#22743);
#6176=VERTEX_POINT('',#22745);
#6177=VERTEX_POINT('',#22747);
#6178=VERTEX_POINT('',#22749);
#6179=VERTEX_POINT('',#22751);
#6180=VERTEX_POINT('',#22755);
#6181=VERTEX_POINT('',#22760);
#6182=VERTEX_POINT('',#22762);
#6183=VERTEX_POINT('',#22763);
#6184=VERTEX_POINT('',#22765);
#6185=VERTEX_POINT('',#22767);
#6186=VERTEX_POINT('',#22769);
#6187=VERTEX_POINT('',#22771);
#6188=VERTEX_POINT('',#22773);
#6189=VERTEX_POINT('',#22775);
#6190=VERTEX_POINT('',#22777);
#6191=VERTEX_POINT('',#22779);
#6192=VERTEX_POINT('',#22781);
#6193=VERTEX_POINT('',#22783);
#6194=VERTEX_POINT('',#22785);
#6195=VERTEX_POINT('',#22787);
#6196=VERTEX_POINT('',#22789);
#6197=VERTEX_POINT('',#22791);
#6198=VERTEX_POINT('',#22793);
#6199=VERTEX_POINT('',#22795);
#6200=VERTEX_POINT('',#22797);
#6201=VERTEX_POINT('',#22799);
#6202=VERTEX_POINT('',#22801);
#6203=VERTEX_POINT('',#22803);
#6204=VERTEX_POINT('',#22805);
#6205=VERTEX_POINT('',#22807);
#6206=VERTEX_POINT('',#22809);
#6207=VERTEX_POINT('',#22811);
#6208=VERTEX_POINT('',#22813);
#6209=VERTEX_POINT('',#22815);
#6210=VERTEX_POINT('',#22817);
#6211=VERTEX_POINT('',#22819);
#6212=VERTEX_POINT('',#22821);
#6213=VERTEX_POINT('',#22823);
#6214=VERTEX_POINT('',#22825);
#6215=VERTEX_POINT('',#22827);
#6216=VERTEX_POINT('',#22829);
#6217=VERTEX_POINT('',#22831);
#6218=VERTEX_POINT('',#22833);
#6219=VERTEX_POINT('',#22835);
#6220=VERTEX_POINT('',#22837);
#6221=VERTEX_POINT('',#22839);
#6222=VERTEX_POINT('',#22841);
#6223=VERTEX_POINT('',#22843);
#6224=VERTEX_POINT('',#22845);
#6225=VERTEX_POINT('',#22847);
#6226=VERTEX_POINT('',#22849);
#6227=VERTEX_POINT('',#22851);
#6228=VERTEX_POINT('',#22853);
#6229=VERTEX_POINT('',#22855);
#6230=VERTEX_POINT('',#22857);
#6231=VERTEX_POINT('',#22859);
#6232=VERTEX_POINT('',#22861);
#6233=VERTEX_POINT('',#22863);
#6234=VERTEX_POINT('',#22865);
#6235=VERTEX_POINT('',#22867);
#6236=VERTEX_POINT('',#22869);
#6237=VERTEX_POINT('',#22871);
#6238=VERTEX_POINT('',#22873);
#6239=VERTEX_POINT('',#22875);
#6240=VERTEX_POINT('',#22877);
#6241=VERTEX_POINT('',#22879);
#6242=VERTEX_POINT('',#22881);
#6243=VERTEX_POINT('',#22883);
#6244=VERTEX_POINT('',#22885);
#6245=VERTEX_POINT('',#22887);
#6246=VERTEX_POINT('',#22889);
#6247=VERTEX_POINT('',#22891);
#6248=VERTEX_POINT('',#22893);
#6249=VERTEX_POINT('',#22895);
#6250=VERTEX_POINT('',#22897);
#6251=VERTEX_POINT('',#22899);
#6252=VERTEX_POINT('',#22901);
#6253=VERTEX_POINT('',#22903);
#6254=VERTEX_POINT('',#22905);
#6255=VERTEX_POINT('',#22907);
#6256=VERTEX_POINT('',#22909);
#6257=VERTEX_POINT('',#22911);
#6258=VERTEX_POINT('',#22913);
#6259=VERTEX_POINT('',#22915);
#6260=VERTEX_POINT('',#22917);
#6261=VERTEX_POINT('',#22919);
#6262=VERTEX_POINT('',#22923);
#7557=EDGE_CURVE('',#6073,#6074,#553,.T.);
#7558=EDGE_CURVE('',#6075,#6073,#554,.T.);
#7559=EDGE_CURVE('',#6074,#6075,#555,.T.);
#7560=EDGE_CURVE('',#6074,#6076,#3569,.T.);
#7561=EDGE_CURVE('',#6077,#6076,#556,.T.);
#7562=EDGE_CURVE('',#6078,#6077,#557,.T.);
#7563=EDGE_CURVE('',#6079,#6078,#558,.T.);
#7564=EDGE_CURVE('',#6076,#6079,#559,.T.);
#7565=EDGE_CURVE('',#6080,#6081,#560,.T.);
#7566=EDGE_CURVE('',#6081,#6080,#561,.T.);
#7567=EDGE_CURVE('',#6081,#6082,#3570,.T.);
#7568=EDGE_CURVE('',#6083,#6082,#562,.T.);
#7569=EDGE_CURVE('',#6084,#6083,#563,.T.);
#7570=EDGE_CURVE('',#6082,#6084,#564,.T.);
#7571=EDGE_CURVE('',#6085,#6085,#5036,.T.);
#7572=EDGE_CURVE('',#6085,#6075,#3571,.T.);
#7573=EDGE_CURVE('',#6073,#6086,#3572,.T.);
#7574=EDGE_CURVE('',#6086,#6086,#5037,.T.);
#7575=EDGE_CURVE('',#6087,#6088,#565,.T.);
#7576=EDGE_CURVE('',#6088,#6089,#566,.T.);
#7577=EDGE_CURVE('',#6089,#6087,#567,.T.);
#7578=EDGE_CURVE('',#6090,#6091,#568,.T.);
#7579=EDGE_CURVE('',#6091,#6092,#569,.T.);
#7580=EDGE_CURVE('',#6092,#6090,#570,.T.);
#7581=EDGE_CURVE('',#6089,#6093,#3573,.T.);
#7582=EDGE_CURVE('',#6094,#6093,#571,.T.);
#7583=EDGE_CURVE('',#6093,#6094,#572,.T.);
#7584=EDGE_CURVE('',#6095,#6096,#573,.T.);
#7585=EDGE_CURVE('',#6096,#6095,#574,.T.);
#7586=EDGE_CURVE('',#6096,#6092,#3574,.T.);
#7587=EDGE_CURVE('',#6097,#6097,#5038,.T.);
#7588=EDGE_CURVE('',#6097,#6077,#3575,.T.);
#7589=EDGE_CURVE('',#6079,#6098,#3576,.T.);
#7590=EDGE_CURVE('',#6098,#6098,#5039,.T.);
#7591=EDGE_CURVE('',#6099,#6099,#5040,.T.);
#7592=EDGE_CURVE('',#6100,#6101,#5041,.T.);
#7593=EDGE_CURVE('',#6102,#6101,#5042,.T.);
#7594=EDGE_CURVE('',#6102,#6103,#5043,.T.);
#7595=EDGE_CURVE('',#6104,#6103,#5044,.T.);
#7596=EDGE_CURVE('',#6104,#6105,#5045,.T.);
#7597=EDGE_CURVE('',#6106,#6105,#5046,.T.);
#7598=EDGE_CURVE('',#6106,#6107,#5047,.T.);
#7599=EDGE_CURVE('',#6108,#6107,#5048,.T.);
#7600=EDGE_CURVE('',#6108,#6109,#5049,.T.);
#7601=EDGE_CURVE('',#6110,#6109,#5050,.T.);
#7602=EDGE_CURVE('',#6110,#6111,#5051,.T.);
#7603=EDGE_CURVE('',#6112,#6111,#5052,.T.);
#7604=EDGE_CURVE('',#6112,#6113,#5053,.T.);
#7605=EDGE_CURVE('',#6114,#6113,#5054,.T.);
#7606=EDGE_CURVE('',#6114,#6115,#5055,.T.);
#7607=EDGE_CURVE('',#6116,#6115,#5056,.T.);
#7608=EDGE_CURVE('',#6116,#6117,#5057,.T.);
#7609=EDGE_CURVE('',#6118,#6117,#5058,.T.);
#7610=EDGE_CURVE('',#6118,#6119,#5059,.T.);
#7611=EDGE_CURVE('',#6120,#6119,#5060,.T.);
#7612=EDGE_CURVE('',#6120,#6121,#5061,.T.);
#7613=EDGE_CURVE('',#6122,#6121,#5062,.T.);
#7614=EDGE_CURVE('',#6122,#6123,#5063,.T.);
#7615=EDGE_CURVE('',#6124,#6123,#5064,.T.);
#7616=EDGE_CURVE('',#6124,#6125,#5065,.T.);
#7617=EDGE_CURVE('',#6126,#6125,#5066,.T.);
#7618=EDGE_CURVE('',#6126,#6127,#5067,.T.);
#7619=EDGE_CURVE('',#6128,#6127,#5068,.T.);
#7620=EDGE_CURVE('',#6128,#6129,#5069,.T.);
#7621=EDGE_CURVE('',#6130,#6129,#5070,.T.);
#7622=EDGE_CURVE('',#6130,#6131,#5071,.T.);
#7623=EDGE_CURVE('',#6132,#6131,#5072,.T.);
#7624=EDGE_CURVE('',#6132,#6133,#5073,.T.);
#7625=EDGE_CURVE('',#6134,#6133,#5074,.T.);
#7626=EDGE_CURVE('',#6134,#6135,#5075,.T.);
#7627=EDGE_CURVE('',#6136,#6135,#5076,.T.);
#7628=EDGE_CURVE('',#6136,#6137,#5077,.T.);
#7629=EDGE_CURVE('',#6138,#6137,#5078,.T.);
#7630=EDGE_CURVE('',#6138,#6139,#5079,.T.);
#7631=EDGE_CURVE('',#6140,#6139,#5080,.T.);
#7632=EDGE_CURVE('',#6140,#6141,#5081,.T.);
#7633=EDGE_CURVE('',#6142,#6141,#5082,.T.);
#7634=EDGE_CURVE('',#6142,#6143,#5083,.T.);
#7635=EDGE_CURVE('',#6144,#6143,#5084,.T.);
#7636=EDGE_CURVE('',#6144,#6145,#5085,.T.);
#7637=EDGE_CURVE('',#6146,#6145,#5086,.T.);
#7638=EDGE_CURVE('',#6146,#6147,#5087,.T.);
#7639=EDGE_CURVE('',#6148,#6147,#5088,.T.);
#7640=EDGE_CURVE('',#6148,#6149,#5089,.T.);
#7641=EDGE_CURVE('',#6150,#6149,#5090,.T.);
#7642=EDGE_CURVE('',#6150,#6151,#5091,.T.);
#7643=EDGE_CURVE('',#6152,#6151,#5092,.T.);
#7644=EDGE_CURVE('',#6152,#6153,#5093,.T.);
#7645=EDGE_CURVE('',#6154,#6153,#5094,.T.);
#7646=EDGE_CURVE('',#6154,#6155,#5095,.T.);
#7647=EDGE_CURVE('',#6156,#6155,#5096,.T.);
#7648=EDGE_CURVE('',#6156,#6157,#5097,.T.);
#7649=EDGE_CURVE('',#6158,#6157,#5098,.T.);
#7650=EDGE_CURVE('',#6158,#6159,#5099,.T.);
#7651=EDGE_CURVE('',#6160,#6159,#5100,.T.);
#7652=EDGE_CURVE('',#6160,#6161,#5101,.T.);
#7653=EDGE_CURVE('',#6162,#6161,#5102,.T.);
#7654=EDGE_CURVE('',#6162,#6163,#5103,.T.);
#7655=EDGE_CURVE('',#6164,#6163,#5104,.T.);
#7656=EDGE_CURVE('',#6164,#6165,#5105,.T.);
#7657=EDGE_CURVE('',#6166,#6165,#5106,.T.);
#7658=EDGE_CURVE('',#6166,#6167,#5107,.T.);
#7659=EDGE_CURVE('',#6168,#6167,#5108,.T.);
#7660=EDGE_CURVE('',#6168,#6169,#5109,.T.);
#7661=EDGE_CURVE('',#6170,#6169,#5110,.T.);
#7662=EDGE_CURVE('',#6170,#6171,#5111,.T.);
#7663=EDGE_CURVE('',#6172,#6171,#5112,.T.);
#7664=EDGE_CURVE('',#6172,#6173,#5113,.T.);
#7665=EDGE_CURVE('',#6174,#6173,#5114,.T.);
#7666=EDGE_CURVE('',#6174,#6175,#5115,.T.);
#7667=EDGE_CURVE('',#6176,#6175,#5116,.T.);
#7668=EDGE_CURVE('',#6176,#6177,#5117,.T.);
#7669=EDGE_CURVE('',#6178,#6177,#5118,.T.);
#7670=EDGE_CURVE('',#6178,#6179,#5119,.T.);
#7671=EDGE_CURVE('',#6100,#6179,#5120,.T.);
#7672=EDGE_CURVE('',#6180,#6180,#5121,.T.);
#7673=EDGE_CURVE('',#6180,#6099,#3577,.T.);
#7674=EDGE_CURVE('',#6181,#6181,#5122,.T.);
#7675=EDGE_CURVE('',#6182,#6183,#5123,.T.);
#7676=EDGE_CURVE('',#6183,#6184,#5124,.T.);
#7677=EDGE_CURVE('',#6184,#6185,#5125,.T.);
#7678=EDGE_CURVE('',#6185,#6186,#5126,.T.);
#7679=EDGE_CURVE('',#6186,#6187,#5127,.T.);
#7680=EDGE_CURVE('',#6187,#6188,#5128,.T.);
#7681=EDGE_CURVE('',#6188,#6189,#5129,.T.);
#7682=EDGE_CURVE('',#6189,#6190,#5130,.T.);
#7683=EDGE_CURVE('',#6190,#6191,#5131,.T.);
#7684=EDGE_CURVE('',#6191,#6192,#5132,.T.);
#7685=EDGE_CURVE('',#6192,#6193,#5133,.T.);
#7686=EDGE_CURVE('',#6193,#6194,#5134,.T.);
#7687=EDGE_CURVE('',#6194,#6195,#5135,.T.);
#7688=EDGE_CURVE('',#6195,#6196,#5136,.T.);
#7689=EDGE_CURVE('',#6196,#6197,#5137,.T.);
#7690=EDGE_CURVE('',#6197,#6198,#5138,.T.);
#7691=EDGE_CURVE('',#6198,#6199,#5139,.T.);
#7692=EDGE_CURVE('',#6199,#6200,#5140,.T.);
#7693=EDGE_CURVE('',#6200,#6201,#5141,.T.);
#7694=EDGE_CURVE('',#6201,#6202,#5142,.T.);
#7695=EDGE_CURVE('',#6202,#6203,#5143,.T.);
#7696=EDGE_CURVE('',#6203,#6204,#5144,.T.);
#7697=EDGE_CURVE('',#6204,#6205,#5145,.T.);
#7698=EDGE_CURVE('',#6205,#6206,#5146,.T.);
#7699=EDGE_CURVE('',#6206,#6207,#5147,.T.);
#7700=EDGE_CURVE('',#6207,#6208,#5148,.T.);
#7701=EDGE_CURVE('',#6208,#6209,#5149,.T.);
#7702=EDGE_CURVE('',#6209,#6210,#5150,.T.);
#7703=EDGE_CURVE('',#6210,#6211,#5151,.T.);
#7704=EDGE_CURVE('',#6211,#6212,#5152,.T.);
#7705=EDGE_CURVE('',#6212,#6213,#5153,.T.);
#7706=EDGE_CURVE('',#6213,#6214,#5154,.T.);
#7707=EDGE_CURVE('',#6214,#6215,#5155,.T.);
#7708=EDGE_CURVE('',#6215,#6216,#5156,.T.);
#7709=EDGE_CURVE('',#6216,#6217,#5157,.T.);
#7710=EDGE_CURVE('',#6217,#6218,#5158,.T.);
#7711=EDGE_CURVE('',#6218,#6219,#5159,.T.);
#7712=EDGE_CURVE('',#6219,#6220,#5160,.T.);
#7713=EDGE_CURVE('',#6220,#6221,#5161,.T.);
#7714=EDGE_CURVE('',#6221,#6222,#5162,.T.);
#7715=EDGE_CURVE('',#6222,#6223,#5163,.T.);
#7716=EDGE_CURVE('',#6223,#6224,#5164,.T.);
#7717=EDGE_CURVE('',#6224,#6225,#5165,.T.);
#7718=EDGE_CURVE('',#6225,#6226,#5166,.T.);
#7719=EDGE_CURVE('',#6226,#6227,#5167,.T.);
#7720=EDGE_CURVE('',#6227,#6228,#5168,.T.);
#7721=EDGE_CURVE('',#6228,#6229,#5169,.T.);
#7722=EDGE_CURVE('',#6229,#6230,#5170,.T.);
#7723=EDGE_CURVE('',#6230,#6231,#5171,.T.);
#7724=EDGE_CURVE('',#6231,#6232,#5172,.T.);
#7725=EDGE_CURVE('',#6232,#6233,#5173,.T.);
#7726=EDGE_CURVE('',#6233,#6234,#5174,.T.);
#7727=EDGE_CURVE('',#6234,#6235,#5175,.T.);
#7728=EDGE_CURVE('',#6235,#6236,#5176,.T.);
#7729=EDGE_CURVE('',#6236,#6237,#5177,.T.);
#7730=EDGE_CURVE('',#6237,#6238,#5178,.T.);
#7731=EDGE_CURVE('',#6238,#6239,#5179,.T.);
#7732=EDGE_CURVE('',#6239,#6240,#5180,.T.);
#7733=EDGE_CURVE('',#6240,#6241,#5181,.T.);
#7734=EDGE_CURVE('',#6241,#6242,#5182,.T.);
#7735=EDGE_CURVE('',#6242,#6243,#5183,.T.);
#7736=EDGE_CURVE('',#6243,#6244,#5184,.T.);
#7737=EDGE_CURVE('',#6244,#6245,#5185,.T.);
#7738=EDGE_CURVE('',#6245,#6246,#5186,.T.);
#7739=EDGE_CURVE('',#6246,#6247,#5187,.T.);
#7740=EDGE_CURVE('',#6247,#6248,#5188,.T.);
#7741=EDGE_CURVE('',#6248,#6249,#5189,.T.);
#7742=EDGE_CURVE('',#6249,#6250,#5190,.T.);
#7743=EDGE_CURVE('',#6250,#6251,#5191,.T.);
#7744=EDGE_CURVE('',#6251,#6252,#5192,.T.);
#7745=EDGE_CURVE('',#6252,#6253,#5193,.T.);
#7746=EDGE_CURVE('',#6253,#6254,#5194,.T.);
#7747=EDGE_CURVE('',#6254,#6255,#5195,.T.);
#7748=EDGE_CURVE('',#6255,#6256,#5196,.T.);
#7749=EDGE_CURVE('',#6256,#6257,#5197,.T.);
#7750=EDGE_CURVE('',#6257,#6258,#5198,.T.);
#7751=EDGE_CURVE('',#6258,#6259,#5199,.T.);
#7752=EDGE_CURVE('',#6259,#6260,#5200,.T.);
#7753=EDGE_CURVE('',#6260,#6261,#5201,.T.);
#7754=EDGE_CURVE('',#6261,#6182,#5202,.T.);
#7755=EDGE_CURVE('',#6262,#6262,#5203,.T.);
#7756=EDGE_CURVE('',#6262,#6181,#3578,.T.);
#7757=EDGE_CURVE('',#6183,#6100,#3579,.T.);
#7758=EDGE_CURVE('',#6101,#6182,#3580,.T.);
#7759=EDGE_CURVE('',#6261,#6102,#3581,.T.);
#7760=EDGE_CURVE('',#6103,#6260,#3582,.T.);
#7761=EDGE_CURVE('',#6259,#6104,#3583,.T.);
#7762=EDGE_CURVE('',#6105,#6258,#3584,.T.);
#7763=EDGE_CURVE('',#6257,#6106,#3585,.T.);
#7764=EDGE_CURVE('',#6107,#6256,#3586,.T.);
#7765=EDGE_CURVE('',#6255,#6108,#3587,.T.);
#7766=EDGE_CURVE('',#6109,#6254,#3588,.T.);
#7767=EDGE_CURVE('',#6253,#6110,#3589,.T.);
#7768=EDGE_CURVE('',#6111,#6252,#3590,.T.);
#7769=EDGE_CURVE('',#6251,#6112,#3591,.T.);
#7770=EDGE_CURVE('',#6113,#6250,#3592,.T.);
#7771=EDGE_CURVE('',#6249,#6114,#3593,.T.);
#7772=EDGE_CURVE('',#6115,#6248,#3594,.T.);
#7773=EDGE_CURVE('',#6247,#6116,#3595,.T.);
#7774=EDGE_CURVE('',#6117,#6246,#3596,.T.);
#7775=EDGE_CURVE('',#6245,#6118,#3597,.T.);
#7776=EDGE_CURVE('',#6119,#6244,#3598,.T.);
#7777=EDGE_CURVE('',#6243,#6120,#3599,.T.);
#7778=EDGE_CURVE('',#6121,#6242,#3600,.T.);
#7779=EDGE_CURVE('',#6241,#6122,#3601,.T.);
#7780=EDGE_CURVE('',#6123,#6240,#3602,.T.);
#7781=EDGE_CURVE('',#6239,#6124,#3603,.T.);
#7782=EDGE_CURVE('',#6125,#6238,#3604,.T.);
#7783=EDGE_CURVE('',#6237,#6126,#3605,.T.);
#7784=EDGE_CURVE('',#6127,#6236,#3606,.T.);
#7785=EDGE_CURVE('',#6235,#6128,#3607,.T.);
#7786=EDGE_CURVE('',#6129,#6234,#3608,.T.);
#7787=EDGE_CURVE('',#6233,#6130,#3609,.T.);
#7788=EDGE_CURVE('',#6131,#6232,#3610,.T.);
#7789=EDGE_CURVE('',#6231,#6132,#3611,.T.);
#7790=EDGE_CURVE('',#6133,#6230,#3612,.T.);
#7791=EDGE_CURVE('',#6229,#6134,#3613,.T.);
#7792=EDGE_CURVE('',#6135,#6228,#3614,.T.);
#7793=EDGE_CURVE('',#6227,#6136,#3615,.T.);
#7794=EDGE_CURVE('',#6137,#6226,#3616,.T.);
#7795=EDGE_CURVE('',#6225,#6138,#3617,.T.);
#7796=EDGE_CURVE('',#6139,#6224,#3618,.T.);
#7797=EDGE_CURVE('',#6223,#6140,#3619,.T.);
#7798=EDGE_CURVE('',#6141,#6222,#3620,.T.);
#7799=EDGE_CURVE('',#6221,#6142,#3621,.T.);
#7800=EDGE_CURVE('',#6143,#6220,#3622,.T.);
#7801=EDGE_CURVE('',#6219,#6144,#3623,.T.);
#7802=EDGE_CURVE('',#6145,#6218,#3624,.T.);
#7803=EDGE_CURVE('',#6217,#6146,#3625,.T.);
#7804=EDGE_CURVE('',#6147,#6216,#3626,.T.);
#7805=EDGE_CURVE('',#6215,#6148,#3627,.T.);
#7806=EDGE_CURVE('',#6149,#6214,#3628,.T.);
#7807=EDGE_CURVE('',#6213,#6150,#3629,.T.);
#7808=EDGE_CURVE('',#6151,#6212,#3630,.T.);
#7809=EDGE_CURVE('',#6211,#6152,#3631,.T.);
#7810=EDGE_CURVE('',#6153,#6210,#3632,.T.);
#7811=EDGE_CURVE('',#6209,#6154,#3633,.T.);
#7812=EDGE_CURVE('',#6155,#6208,#3634,.T.);
#7813=EDGE_CURVE('',#6207,#6156,#3635,.T.);
#7814=EDGE_CURVE('',#6157,#6206,#3636,.T.);
#7815=EDGE_CURVE('',#6205,#6158,#3637,.T.);
#7816=EDGE_CURVE('',#6159,#6204,#3638,.T.);
#7817=EDGE_CURVE('',#6203,#6160,#3639,.T.);
#7818=EDGE_CURVE('',#6161,#6202,#3640,.T.);
#7819=EDGE_CURVE('',#6201,#6162,#3641,.T.);
#7820=EDGE_CURVE('',#6163,#6200,#3642,.T.);
#7821=EDGE_CURVE('',#6199,#6164,#3643,.T.);
#7822=EDGE_CURVE('',#6165,#6198,#3644,.T.);
#7823=EDGE_CURVE('',#6197,#6166,#3645,.T.);
#7824=EDGE_CURVE('',#6167,#6196,#3646,.T.);
#7825=EDGE_CURVE('',#6195,#6168,#3647,.T.);
#7826=EDGE_CURVE('',#6169,#6194,#3648,.T.);
#7827=EDGE_CURVE('',#6193,#6170,#3649,.T.);
#7828=EDGE_CURVE('',#6171,#6192,#3650,.T.);
#7829=EDGE_CURVE('',#6191,#6172,#3651,.T.);
#7830=EDGE_CURVE('',#6173,#6190,#3652,.T.);
#7831=EDGE_CURVE('',#6189,#6174,#3653,.T.);
#7832=EDGE_CURVE('',#6175,#6188,#3654,.T.);
#7833=EDGE_CURVE('',#6187,#6176,#3655,.T.);
#7834=EDGE_CURVE('',#6177,#6186,#3656,.T.);
#7835=EDGE_CURVE('',#6179,#6184,#3657,.T.);
#7836=EDGE_CURVE('',#6185,#6178,#3658,.T.);
#10396=ORIENTED_EDGE('',*,*,#7557,.F.);
#10397=ORIENTED_EDGE('',*,*,#7558,.F.);
#10398=ORIENTED_EDGE('',*,*,#7559,.F.);
#10399=ORIENTED_EDGE('',*,*,#7560,.T.);
#10400=ORIENTED_EDGE('',*,*,#7561,.F.);
#10401=ORIENTED_EDGE('',*,*,#7562,.F.);
#10402=ORIENTED_EDGE('',*,*,#7563,.F.);
#10403=ORIENTED_EDGE('',*,*,#7564,.F.);
#10404=ORIENTED_EDGE('',*,*,#7560,.F.);
#10405=ORIENTED_EDGE('',*,*,#7565,.F.);
#10406=ORIENTED_EDGE('',*,*,#7566,.F.);
#10407=ORIENTED_EDGE('',*,*,#7567,.T.);
#10408=ORIENTED_EDGE('',*,*,#7568,.F.);
#10409=ORIENTED_EDGE('',*,*,#7569,.F.);
#10410=ORIENTED_EDGE('',*,*,#7570,.F.);
#10411=ORIENTED_EDGE('',*,*,#7567,.F.);
#10412=ORIENTED_EDGE('',*,*,#7571,.F.);
#10413=ORIENTED_EDGE('',*,*,#7572,.T.);
#10414=ORIENTED_EDGE('',*,*,#7558,.T.);
#10415=ORIENTED_EDGE('',*,*,#7573,.T.);
#10416=ORIENTED_EDGE('',*,*,#7574,.F.);
#10417=ORIENTED_EDGE('',*,*,#7573,.F.);
#10418=ORIENTED_EDGE('',*,*,#7557,.T.);
#10419=ORIENTED_EDGE('',*,*,#7559,.T.);
#10420=ORIENTED_EDGE('',*,*,#7572,.F.);
#10421=ORIENTED_EDGE('',*,*,#7569,.T.);
#10422=ORIENTED_EDGE('',*,*,#7568,.T.);
#10423=ORIENTED_EDGE('',*,*,#7570,.T.);
#10424=ORIENTED_EDGE('',*,*,#7575,.T.);
#10425=ORIENTED_EDGE('',*,*,#7576,.T.);
#10426=ORIENTED_EDGE('',*,*,#7577,.T.);
#10427=ORIENTED_EDGE('',*,*,#7578,.T.);
#10428=ORIENTED_EDGE('',*,*,#7579,.T.);
#10429=ORIENTED_EDGE('',*,*,#7580,.T.);
#10430=ORIENTED_EDGE('',*,*,#7576,.F.);
#10431=ORIENTED_EDGE('',*,*,#7575,.F.);
#10432=ORIENTED_EDGE('',*,*,#7577,.F.);
#10433=ORIENTED_EDGE('',*,*,#7581,.T.);
#10434=ORIENTED_EDGE('',*,*,#7582,.F.);
#10435=ORIENTED_EDGE('',*,*,#7583,.F.);
#10436=ORIENTED_EDGE('',*,*,#7581,.F.);
#10437=ORIENTED_EDGE('',*,*,#7584,.F.);
#10438=ORIENTED_EDGE('',*,*,#7585,.F.);
#10439=ORIENTED_EDGE('',*,*,#7586,.T.);
#10440=ORIENTED_EDGE('',*,*,#7579,.F.);
#10441=ORIENTED_EDGE('',*,*,#7578,.F.);
#10442=ORIENTED_EDGE('',*,*,#7580,.F.);
#10443=ORIENTED_EDGE('',*,*,#7586,.F.);
#10444=ORIENTED_EDGE('',*,*,#7587,.F.);
#10445=ORIENTED_EDGE('',*,*,#7588,.T.);
#10446=ORIENTED_EDGE('',*,*,#7561,.T.);
#10447=ORIENTED_EDGE('',*,*,#7564,.T.);
#10448=ORIENTED_EDGE('',*,*,#7589,.T.);
#10449=ORIENTED_EDGE('',*,*,#7590,.F.);
#10450=ORIENTED_EDGE('',*,*,#7589,.F.);
#10451=ORIENTED_EDGE('',*,*,#7563,.T.);
#10452=ORIENTED_EDGE('',*,*,#7562,.T.);
#10453=ORIENTED_EDGE('',*,*,#7588,.F.);
#10454=ORIENTED_EDGE('',*,*,#7565,.T.);
#10455=ORIENTED_EDGE('',*,*,#7566,.T.);
#10456=ORIENTED_EDGE('',*,*,#7584,.T.);
#10457=ORIENTED_EDGE('',*,*,#7585,.T.);
#10458=ORIENTED_EDGE('',*,*,#7582,.T.);
#10459=ORIENTED_EDGE('',*,*,#7583,.T.);
#10460=ORIENTED_EDGE('',*,*,#7571,.T.);
#10461=ORIENTED_EDGE('',*,*,#7587,.T.);
#10462=ORIENTED_EDGE('',*,*,#7591,.T.);
#10463=ORIENTED_EDGE('',*,*,#7592,.T.);
#10464=ORIENTED_EDGE('',*,*,#7593,.F.);
#10465=ORIENTED_EDGE('',*,*,#7594,.T.);
#10466=ORIENTED_EDGE('',*,*,#7595,.F.);
#10467=ORIENTED_EDGE('',*,*,#7596,.T.);
#10468=ORIENTED_EDGE('',*,*,#7597,.F.);
#10469=ORIENTED_EDGE('',*,*,#7598,.T.);
#10470=ORIENTED_EDGE('',*,*,#7599,.F.);
#10471=ORIENTED_EDGE('',*,*,#7600,.T.);
#10472=ORIENTED_EDGE('',*,*,#7601,.F.);
#10473=ORIENTED_EDGE('',*,*,#7602,.T.);
#10474=ORIENTED_EDGE('',*,*,#7603,.F.);
#10475=ORIENTED_EDGE('',*,*,#7604,.T.);
#10476=ORIENTED_EDGE('',*,*,#7605,.F.);
#10477=ORIENTED_EDGE('',*,*,#7606,.T.);
#10478=ORIENTED_EDGE('',*,*,#7607,.F.);
#10479=ORIENTED_EDGE('',*,*,#7608,.T.);
#10480=ORIENTED_EDGE('',*,*,#7609,.F.);
#10481=ORIENTED_EDGE('',*,*,#7610,.T.);
#10482=ORIENTED_EDGE('',*,*,#7611,.F.);
#10483=ORIENTED_EDGE('',*,*,#7612,.T.);
#10484=ORIENTED_EDGE('',*,*,#7613,.F.);
#10485=ORIENTED_EDGE('',*,*,#7614,.T.);
#10486=ORIENTED_EDGE('',*,*,#7615,.F.);
#10487=ORIENTED_EDGE('',*,*,#7616,.T.);
#10488=ORIENTED_EDGE('',*,*,#7617,.F.);
#10489=ORIENTED_EDGE('',*,*,#7618,.T.);
#10490=ORIENTED_EDGE('',*,*,#7619,.F.);
#10491=ORIENTED_EDGE('',*,*,#7620,.T.);
#10492=ORIENTED_EDGE('',*,*,#7621,.F.);
#10493=ORIENTED_EDGE('',*,*,#7622,.T.);
#10494=ORIENTED_EDGE('',*,*,#7623,.F.);
#10495=ORIENTED_EDGE('',*,*,#7624,.T.);
#10496=ORIENTED_EDGE('',*,*,#7625,.F.);
#10497=ORIENTED_EDGE('',*,*,#7626,.T.);
#10498=ORIENTED_EDGE('',*,*,#7627,.F.);
#10499=ORIENTED_EDGE('',*,*,#7628,.T.);
#10500=ORIENTED_EDGE('',*,*,#7629,.F.);
#10501=ORIENTED_EDGE('',*,*,#7630,.T.);
#10502=ORIENTED_EDGE('',*,*,#7631,.F.);
#10503=ORIENTED_EDGE('',*,*,#7632,.T.);
#10504=ORIENTED_EDGE('',*,*,#7633,.F.);
#10505=ORIENTED_EDGE('',*,*,#7634,.T.);
#10506=ORIENTED_EDGE('',*,*,#7635,.F.);
#10507=ORIENTED_EDGE('',*,*,#7636,.T.);
#10508=ORIENTED_EDGE('',*,*,#7637,.F.);
#10509=ORIENTED_EDGE('',*,*,#7638,.T.);
#10510=ORIENTED_EDGE('',*,*,#7639,.F.);
#10511=ORIENTED_EDGE('',*,*,#7640,.T.);
#10512=ORIENTED_EDGE('',*,*,#7641,.F.);
#10513=ORIENTED_EDGE('',*,*,#7642,.T.);
#10514=ORIENTED_EDGE('',*,*,#7643,.F.);
#10515=ORIENTED_EDGE('',*,*,#7644,.T.);
#10516=ORIENTED_EDGE('',*,*,#7645,.F.);
#10517=ORIENTED_EDGE('',*,*,#7646,.T.);
#10518=ORIENTED_EDGE('',*,*,#7647,.F.);
#10519=ORIENTED_EDGE('',*,*,#7648,.T.);
#10520=ORIENTED_EDGE('',*,*,#7649,.F.);
#10521=ORIENTED_EDGE('',*,*,#7650,.T.);
#10522=ORIENTED_EDGE('',*,*,#7651,.F.);
#10523=ORIENTED_EDGE('',*,*,#7652,.T.);
#10524=ORIENTED_EDGE('',*,*,#7653,.F.);
#10525=ORIENTED_EDGE('',*,*,#7654,.T.);
#10526=ORIENTED_EDGE('',*,*,#7655,.F.);
#10527=ORIENTED_EDGE('',*,*,#7656,.T.);
#10528=ORIENTED_EDGE('',*,*,#7657,.F.);
#10529=ORIENTED_EDGE('',*,*,#7658,.T.);
#10530=ORIENTED_EDGE('',*,*,#7659,.F.);
#10531=ORIENTED_EDGE('',*,*,#7660,.T.);
#10532=ORIENTED_EDGE('',*,*,#7661,.F.);
#10533=ORIENTED_EDGE('',*,*,#7662,.T.);
#10534=ORIENTED_EDGE('',*,*,#7663,.F.);
#10535=ORIENTED_EDGE('',*,*,#7664,.T.);
#10536=ORIENTED_EDGE('',*,*,#7665,.F.);
#10537=ORIENTED_EDGE('',*,*,#7666,.T.);
#10538=ORIENTED_EDGE('',*,*,#7667,.F.);
#10539=ORIENTED_EDGE('',*,*,#7668,.T.);
#10540=ORIENTED_EDGE('',*,*,#7669,.F.);
#10541=ORIENTED_EDGE('',*,*,#7670,.T.);
#10542=ORIENTED_EDGE('',*,*,#7671,.F.);
#10543=ORIENTED_EDGE('',*,*,#7672,.F.);
#10544=ORIENTED_EDGE('',*,*,#7673,.T.);
#10545=ORIENTED_EDGE('',*,*,#7591,.F.);
#10546=ORIENTED_EDGE('',*,*,#7673,.F.);
#10547=ORIENTED_EDGE('',*,*,#7672,.T.);
#10548=ORIENTED_EDGE('',*,*,#7574,.T.);
#10549=ORIENTED_EDGE('',*,*,#7674,.F.);
#10550=ORIENTED_EDGE('',*,*,#7675,.T.);
#10551=ORIENTED_EDGE('',*,*,#7676,.T.);
#10552=ORIENTED_EDGE('',*,*,#7677,.T.);
#10553=ORIENTED_EDGE('',*,*,#7678,.T.);
#10554=ORIENTED_EDGE('',*,*,#7679,.T.);
#10555=ORIENTED_EDGE('',*,*,#7680,.T.);
#10556=ORIENTED_EDGE('',*,*,#7681,.T.);
#10557=ORIENTED_EDGE('',*,*,#7682,.T.);
#10558=ORIENTED_EDGE('',*,*,#7683,.T.);
#10559=ORIENTED_EDGE('',*,*,#7684,.T.);
#10560=ORIENTED_EDGE('',*,*,#7685,.T.);
#10561=ORIENTED_EDGE('',*,*,#7686,.T.);
#10562=ORIENTED_EDGE('',*,*,#7687,.T.);
#10563=ORIENTED_EDGE('',*,*,#7688,.T.);
#10564=ORIENTED_EDGE('',*,*,#7689,.T.);
#10565=ORIENTED_EDGE('',*,*,#7690,.T.);
#10566=ORIENTED_EDGE('',*,*,#7691,.T.);
#10567=ORIENTED_EDGE('',*,*,#7692,.T.);
#10568=ORIENTED_EDGE('',*,*,#7693,.T.);
#10569=ORIENTED_EDGE('',*,*,#7694,.T.);
#10570=ORIENTED_EDGE('',*,*,#7695,.T.);
#10571=ORIENTED_EDGE('',*,*,#7696,.T.);
#10572=ORIENTED_EDGE('',*,*,#7697,.T.);
#10573=ORIENTED_EDGE('',*,*,#7698,.T.);
#10574=ORIENTED_EDGE('',*,*,#7699,.T.);
#10575=ORIENTED_EDGE('',*,*,#7700,.T.);
#10576=ORIENTED_EDGE('',*,*,#7701,.T.);
#10577=ORIENTED_EDGE('',*,*,#7702,.T.);
#10578=ORIENTED_EDGE('',*,*,#7703,.T.);
#10579=ORIENTED_EDGE('',*,*,#7704,.T.);
#10580=ORIENTED_EDGE('',*,*,#7705,.T.);
#10581=ORIENTED_EDGE('',*,*,#7706,.T.);
#10582=ORIENTED_EDGE('',*,*,#7707,.T.);
#10583=ORIENTED_EDGE('',*,*,#7708,.T.);
#10584=ORIENTED_EDGE('',*,*,#7709,.T.);
#10585=ORIENTED_EDGE('',*,*,#7710,.T.);
#10586=ORIENTED_EDGE('',*,*,#7711,.T.);
#10587=ORIENTED_EDGE('',*,*,#7712,.T.);
#10588=ORIENTED_EDGE('',*,*,#7713,.T.);
#10589=ORIENTED_EDGE('',*,*,#7714,.T.);
#10590=ORIENTED_EDGE('',*,*,#7715,.T.);
#10591=ORIENTED_EDGE('',*,*,#7716,.T.);
#10592=ORIENTED_EDGE('',*,*,#7717,.T.);
#10593=ORIENTED_EDGE('',*,*,#7718,.T.);
#10594=ORIENTED_EDGE('',*,*,#7719,.T.);
#10595=ORIENTED_EDGE('',*,*,#7720,.T.);
#10596=ORIENTED_EDGE('',*,*,#7721,.T.);
#10597=ORIENTED_EDGE('',*,*,#7722,.T.);
#10598=ORIENTED_EDGE('',*,*,#7723,.T.);
#10599=ORIENTED_EDGE('',*,*,#7724,.T.);
#10600=ORIENTED_EDGE('',*,*,#7725,.T.);
#10601=ORIENTED_EDGE('',*,*,#7726,.T.);
#10602=ORIENTED_EDGE('',*,*,#7727,.T.);
#10603=ORIENTED_EDGE('',*,*,#7728,.T.);
#10604=ORIENTED_EDGE('',*,*,#7729,.T.);
#10605=ORIENTED_EDGE('',*,*,#7730,.T.);
#10606=ORIENTED_EDGE('',*,*,#7731,.T.);
#10607=ORIENTED_EDGE('',*,*,#7732,.T.);
#10608=ORIENTED_EDGE('',*,*,#7733,.T.);
#10609=ORIENTED_EDGE('',*,*,#7734,.T.);
#10610=ORIENTED_EDGE('',*,*,#7735,.T.);
#10611=ORIENTED_EDGE('',*,*,#7736,.T.);
#10612=ORIENTED_EDGE('',*,*,#7737,.T.);
#10613=ORIENTED_EDGE('',*,*,#7738,.T.);
#10614=ORIENTED_EDGE('',*,*,#7739,.T.);
#10615=ORIENTED_EDGE('',*,*,#7740,.T.);
#10616=ORIENTED_EDGE('',*,*,#7741,.T.);
#10617=ORIENTED_EDGE('',*,*,#7742,.T.);
#10618=ORIENTED_EDGE('',*,*,#7743,.T.);
#10619=ORIENTED_EDGE('',*,*,#7744,.T.);
#10620=ORIENTED_EDGE('',*,*,#7745,.T.);
#10621=ORIENTED_EDGE('',*,*,#7746,.T.);
#10622=ORIENTED_EDGE('',*,*,#7747,.T.);
#10623=ORIENTED_EDGE('',*,*,#7748,.T.);
#10624=ORIENTED_EDGE('',*,*,#7749,.T.);
#10625=ORIENTED_EDGE('',*,*,#7750,.T.);
#10626=ORIENTED_EDGE('',*,*,#7751,.T.);
#10627=ORIENTED_EDGE('',*,*,#7752,.T.);
#10628=ORIENTED_EDGE('',*,*,#7753,.T.);
#10629=ORIENTED_EDGE('',*,*,#7754,.T.);
#10630=ORIENTED_EDGE('',*,*,#7755,.F.);
#10631=ORIENTED_EDGE('',*,*,#7756,.T.);
#10632=ORIENTED_EDGE('',*,*,#7674,.T.);
#10633=ORIENTED_EDGE('',*,*,#7756,.F.);
#10634=ORIENTED_EDGE('',*,*,#7755,.T.);
#10635=ORIENTED_EDGE('',*,*,#7590,.T.);
#10636=ORIENTED_EDGE('',*,*,#7757,.F.);
#10637=ORIENTED_EDGE('',*,*,#7675,.F.);
#10638=ORIENTED_EDGE('',*,*,#7758,.F.);
#10639=ORIENTED_EDGE('',*,*,#7592,.F.);
#10640=ORIENTED_EDGE('',*,*,#7758,.T.);
#10641=ORIENTED_EDGE('',*,*,#7754,.F.);
#10642=ORIENTED_EDGE('',*,*,#7759,.T.);
#10643=ORIENTED_EDGE('',*,*,#7593,.T.);
#10644=ORIENTED_EDGE('',*,*,#7759,.F.);
#10645=ORIENTED_EDGE('',*,*,#7753,.F.);
#10646=ORIENTED_EDGE('',*,*,#7760,.F.);
#10647=ORIENTED_EDGE('',*,*,#7594,.F.);
#10648=ORIENTED_EDGE('',*,*,#7760,.T.);
#10649=ORIENTED_EDGE('',*,*,#7752,.F.);
#10650=ORIENTED_EDGE('',*,*,#7761,.T.);
#10651=ORIENTED_EDGE('',*,*,#7595,.T.);
#10652=ORIENTED_EDGE('',*,*,#7761,.F.);
#10653=ORIENTED_EDGE('',*,*,#7751,.F.);
#10654=ORIENTED_EDGE('',*,*,#7762,.F.);
#10655=ORIENTED_EDGE('',*,*,#7596,.F.);
#10656=ORIENTED_EDGE('',*,*,#7762,.T.);
#10657=ORIENTED_EDGE('',*,*,#7750,.F.);
#10658=ORIENTED_EDGE('',*,*,#7763,.T.);
#10659=ORIENTED_EDGE('',*,*,#7597,.T.);
#10660=ORIENTED_EDGE('',*,*,#7763,.F.);
#10661=ORIENTED_EDGE('',*,*,#7749,.F.);
#10662=ORIENTED_EDGE('',*,*,#7764,.F.);
#10663=ORIENTED_EDGE('',*,*,#7598,.F.);
#10664=ORIENTED_EDGE('',*,*,#7764,.T.);
#10665=ORIENTED_EDGE('',*,*,#7748,.F.);
#10666=ORIENTED_EDGE('',*,*,#7765,.T.);
#10667=ORIENTED_EDGE('',*,*,#7599,.T.);
#10668=ORIENTED_EDGE('',*,*,#7765,.F.);
#10669=ORIENTED_EDGE('',*,*,#7747,.F.);
#10670=ORIENTED_EDGE('',*,*,#7766,.F.);
#10671=ORIENTED_EDGE('',*,*,#7600,.F.);
#10672=ORIENTED_EDGE('',*,*,#7766,.T.);
#10673=ORIENTED_EDGE('',*,*,#7746,.F.);
#10674=ORIENTED_EDGE('',*,*,#7767,.T.);
#10675=ORIENTED_EDGE('',*,*,#7601,.T.);
#10676=ORIENTED_EDGE('',*,*,#7767,.F.);
#10677=ORIENTED_EDGE('',*,*,#7745,.F.);
#10678=ORIENTED_EDGE('',*,*,#7768,.F.);
#10679=ORIENTED_EDGE('',*,*,#7602,.F.);
#10680=ORIENTED_EDGE('',*,*,#7768,.T.);
#10681=ORIENTED_EDGE('',*,*,#7744,.F.);
#10682=ORIENTED_EDGE('',*,*,#7769,.T.);
#10683=ORIENTED_EDGE('',*,*,#7603,.T.);
#10684=ORIENTED_EDGE('',*,*,#7769,.F.);
#10685=ORIENTED_EDGE('',*,*,#7743,.F.);
#10686=ORIENTED_EDGE('',*,*,#7770,.F.);
#10687=ORIENTED_EDGE('',*,*,#7604,.F.);
#10688=ORIENTED_EDGE('',*,*,#7770,.T.);
#10689=ORIENTED_EDGE('',*,*,#7742,.F.);
#10690=ORIENTED_EDGE('',*,*,#7771,.T.);
#10691=ORIENTED_EDGE('',*,*,#7605,.T.);
#10692=ORIENTED_EDGE('',*,*,#7771,.F.);
#10693=ORIENTED_EDGE('',*,*,#7741,.F.);
#10694=ORIENTED_EDGE('',*,*,#7772,.F.);
#10695=ORIENTED_EDGE('',*,*,#7606,.F.);
#10696=ORIENTED_EDGE('',*,*,#7772,.T.);
#10697=ORIENTED_EDGE('',*,*,#7740,.F.);
#10698=ORIENTED_EDGE('',*,*,#7773,.T.);
#10699=ORIENTED_EDGE('',*,*,#7607,.T.);
#10700=ORIENTED_EDGE('',*,*,#7773,.F.);
#10701=ORIENTED_EDGE('',*,*,#7739,.F.);
#10702=ORIENTED_EDGE('',*,*,#7774,.F.);
#10703=ORIENTED_EDGE('',*,*,#7608,.F.);
#10704=ORIENTED_EDGE('',*,*,#7774,.T.);
#10705=ORIENTED_EDGE('',*,*,#7738,.F.);
#10706=ORIENTED_EDGE('',*,*,#7775,.T.);
#10707=ORIENTED_EDGE('',*,*,#7609,.T.);
#10708=ORIENTED_EDGE('',*,*,#7775,.F.);
#10709=ORIENTED_EDGE('',*,*,#7737,.F.);
#10710=ORIENTED_EDGE('',*,*,#7776,.F.);
#10711=ORIENTED_EDGE('',*,*,#7610,.F.);
#10712=ORIENTED_EDGE('',*,*,#7776,.T.);
#10713=ORIENTED_EDGE('',*,*,#7736,.F.);
#10714=ORIENTED_EDGE('',*,*,#7777,.T.);
#10715=ORIENTED_EDGE('',*,*,#7611,.T.);
#10716=ORIENTED_EDGE('',*,*,#7777,.F.);
#10717=ORIENTED_EDGE('',*,*,#7735,.F.);
#10718=ORIENTED_EDGE('',*,*,#7778,.F.);
#10719=ORIENTED_EDGE('',*,*,#7612,.F.);
#10720=ORIENTED_EDGE('',*,*,#7778,.T.);
#10721=ORIENTED_EDGE('',*,*,#7734,.F.);
#10722=ORIENTED_EDGE('',*,*,#7779,.T.);
#10723=ORIENTED_EDGE('',*,*,#7613,.T.);
#10724=ORIENTED_EDGE('',*,*,#7779,.F.);
#10725=ORIENTED_EDGE('',*,*,#7733,.F.);
#10726=ORIENTED_EDGE('',*,*,#7780,.F.);
#10727=ORIENTED_EDGE('',*,*,#7614,.F.);
#10728=ORIENTED_EDGE('',*,*,#7780,.T.);
#10729=ORIENTED_EDGE('',*,*,#7732,.F.);
#10730=ORIENTED_EDGE('',*,*,#7781,.T.);
#10731=ORIENTED_EDGE('',*,*,#7615,.T.);
#10732=ORIENTED_EDGE('',*,*,#7781,.F.);
#10733=ORIENTED_EDGE('',*,*,#7731,.F.);
#10734=ORIENTED_EDGE('',*,*,#7782,.F.);
#10735=ORIENTED_EDGE('',*,*,#7616,.F.);
#10736=ORIENTED_EDGE('',*,*,#7782,.T.);
#10737=ORIENTED_EDGE('',*,*,#7730,.F.);
#10738=ORIENTED_EDGE('',*,*,#7783,.T.);
#10739=ORIENTED_EDGE('',*,*,#7617,.T.);
#10740=ORIENTED_EDGE('',*,*,#7783,.F.);
#10741=ORIENTED_EDGE('',*,*,#7729,.F.);
#10742=ORIENTED_EDGE('',*,*,#7784,.F.);
#10743=ORIENTED_EDGE('',*,*,#7618,.F.);
#10744=ORIENTED_EDGE('',*,*,#7784,.T.);
#10745=ORIENTED_EDGE('',*,*,#7728,.F.);
#10746=ORIENTED_EDGE('',*,*,#7785,.T.);
#10747=ORIENTED_EDGE('',*,*,#7619,.T.);
#10748=ORIENTED_EDGE('',*,*,#7785,.F.);
#10749=ORIENTED_EDGE('',*,*,#7727,.F.);
#10750=ORIENTED_EDGE('',*,*,#7786,.F.);
#10751=ORIENTED_EDGE('',*,*,#7620,.F.);
#10752=ORIENTED_EDGE('',*,*,#7786,.T.);
#10753=ORIENTED_EDGE('',*,*,#7726,.F.);
#10754=ORIENTED_EDGE('',*,*,#7787,.T.);
#10755=ORIENTED_EDGE('',*,*,#7621,.T.);
#10756=ORIENTED_EDGE('',*,*,#7787,.F.);
#10757=ORIENTED_EDGE('',*,*,#7725,.F.);
#10758=ORIENTED_EDGE('',*,*,#7788,.F.);
#10759=ORIENTED_EDGE('',*,*,#7622,.F.);
#10760=ORIENTED_EDGE('',*,*,#7788,.T.);
#10761=ORIENTED_EDGE('',*,*,#7724,.F.);
#10762=ORIENTED_EDGE('',*,*,#7789,.T.);
#10763=ORIENTED_EDGE('',*,*,#7623,.T.);
#10764=ORIENTED_EDGE('',*,*,#7789,.F.);
#10765=ORIENTED_EDGE('',*,*,#7723,.F.);
#10766=ORIENTED_EDGE('',*,*,#7790,.F.);
#10767=ORIENTED_EDGE('',*,*,#7624,.F.);
#10768=ORIENTED_EDGE('',*,*,#7790,.T.);
#10769=ORIENTED_EDGE('',*,*,#7722,.F.);
#10770=ORIENTED_EDGE('',*,*,#7791,.T.);
#10771=ORIENTED_EDGE('',*,*,#7625,.T.);
#10772=ORIENTED_EDGE('',*,*,#7791,.F.);
#10773=ORIENTED_EDGE('',*,*,#7721,.F.);
#10774=ORIENTED_EDGE('',*,*,#7792,.F.);
#10775=ORIENTED_EDGE('',*,*,#7626,.F.);
#10776=ORIENTED_EDGE('',*,*,#7792,.T.);
#10777=ORIENTED_EDGE('',*,*,#7720,.F.);
#10778=ORIENTED_EDGE('',*,*,#7793,.T.);
#10779=ORIENTED_EDGE('',*,*,#7627,.T.);
#10780=ORIENTED_EDGE('',*,*,#7793,.F.);
#10781=ORIENTED_EDGE('',*,*,#7719,.F.);
#10782=ORIENTED_EDGE('',*,*,#7794,.F.);
#10783=ORIENTED_EDGE('',*,*,#7628,.F.);
#10784=ORIENTED_EDGE('',*,*,#7794,.T.);
#10785=ORIENTED_EDGE('',*,*,#7718,.F.);
#10786=ORIENTED_EDGE('',*,*,#7795,.T.);
#10787=ORIENTED_EDGE('',*,*,#7629,.T.);
#10788=ORIENTED_EDGE('',*,*,#7795,.F.);
#10789=ORIENTED_EDGE('',*,*,#7717,.F.);
#10790=ORIENTED_EDGE('',*,*,#7796,.F.);
#10791=ORIENTED_EDGE('',*,*,#7630,.F.);
#10792=ORIENTED_EDGE('',*,*,#7796,.T.);
#10793=ORIENTED_EDGE('',*,*,#7716,.F.);
#10794=ORIENTED_EDGE('',*,*,#7797,.T.);
#10795=ORIENTED_EDGE('',*,*,#7631,.T.);
#10796=ORIENTED_EDGE('',*,*,#7797,.F.);
#10797=ORIENTED_EDGE('',*,*,#7715,.F.);
#10798=ORIENTED_EDGE('',*,*,#7798,.F.);
#10799=ORIENTED_EDGE('',*,*,#7632,.F.);
#10800=ORIENTED_EDGE('',*,*,#7798,.T.);
#10801=ORIENTED_EDGE('',*,*,#7714,.F.);
#10802=ORIENTED_EDGE('',*,*,#7799,.T.);
#10803=ORIENTED_EDGE('',*,*,#7633,.T.);
#10804=ORIENTED_EDGE('',*,*,#7799,.F.);
#10805=ORIENTED_EDGE('',*,*,#7713,.F.);
#10806=ORIENTED_EDGE('',*,*,#7800,.F.);
#10807=ORIENTED_EDGE('',*,*,#7634,.F.);
#10808=ORIENTED_EDGE('',*,*,#7800,.T.);
#10809=ORIENTED_EDGE('',*,*,#7712,.F.);
#10810=ORIENTED_EDGE('',*,*,#7801,.T.);
#10811=ORIENTED_EDGE('',*,*,#7635,.T.);
#10812=ORIENTED_EDGE('',*,*,#7801,.F.);
#10813=ORIENTED_EDGE('',*,*,#7711,.F.);
#10814=ORIENTED_EDGE('',*,*,#7802,.F.);
#10815=ORIENTED_EDGE('',*,*,#7636,.F.);
#10816=ORIENTED_EDGE('',*,*,#7802,.T.);
#10817=ORIENTED_EDGE('',*,*,#7710,.F.);
#10818=ORIENTED_EDGE('',*,*,#7803,.T.);
#10819=ORIENTED_EDGE('',*,*,#7637,.T.);
#10820=ORIENTED_EDGE('',*,*,#7803,.F.);
#10821=ORIENTED_EDGE('',*,*,#7709,.F.);
#10822=ORIENTED_EDGE('',*,*,#7804,.F.);
#10823=ORIENTED_EDGE('',*,*,#7638,.F.);
#10824=ORIENTED_EDGE('',*,*,#7804,.T.);
#10825=ORIENTED_EDGE('',*,*,#7708,.F.);
#10826=ORIENTED_EDGE('',*,*,#7805,.T.);
#10827=ORIENTED_EDGE('',*,*,#7639,.T.);
#10828=ORIENTED_EDGE('',*,*,#7805,.F.);
#10829=ORIENTED_EDGE('',*,*,#7707,.F.);
#10830=ORIENTED_EDGE('',*,*,#7806,.F.);
#10831=ORIENTED_EDGE('',*,*,#7640,.F.);
#10832=ORIENTED_EDGE('',*,*,#7806,.T.);
#10833=ORIENTED_EDGE('',*,*,#7706,.F.);
#10834=ORIENTED_EDGE('',*,*,#7807,.T.);
#10835=ORIENTED_EDGE('',*,*,#7641,.T.);
#10836=ORIENTED_EDGE('',*,*,#7807,.F.);
#10837=ORIENTED_EDGE('',*,*,#7705,.F.);
#10838=ORIENTED_EDGE('',*,*,#7808,.F.);
#10839=ORIENTED_EDGE('',*,*,#7642,.F.);
#10840=ORIENTED_EDGE('',*,*,#7808,.T.);
#10841=ORIENTED_EDGE('',*,*,#7704,.F.);
#10842=ORIENTED_EDGE('',*,*,#7809,.T.);
#10843=ORIENTED_EDGE('',*,*,#7643,.T.);
#10844=ORIENTED_EDGE('',*,*,#7809,.F.);
#10845=ORIENTED_EDGE('',*,*,#7703,.F.);
#10846=ORIENTED_EDGE('',*,*,#7810,.F.);
#10847=ORIENTED_EDGE('',*,*,#7644,.F.);
#10848=ORIENTED_EDGE('',*,*,#7810,.T.);
#10849=ORIENTED_EDGE('',*,*,#7702,.F.);
#10850=ORIENTED_EDGE('',*,*,#7811,.T.);
#10851=ORIENTED_EDGE('',*,*,#7645,.T.);
#10852=ORIENTED_EDGE('',*,*,#7811,.F.);
#10853=ORIENTED_EDGE('',*,*,#7701,.F.);
#10854=ORIENTED_EDGE('',*,*,#7812,.F.);
#10855=ORIENTED_EDGE('',*,*,#7646,.F.);
#10856=ORIENTED_EDGE('',*,*,#7812,.T.);
#10857=ORIENTED_EDGE('',*,*,#7700,.F.);
#10858=ORIENTED_EDGE('',*,*,#7813,.T.);
#10859=ORIENTED_EDGE('',*,*,#7647,.T.);
#10860=ORIENTED_EDGE('',*,*,#7813,.F.);
#10861=ORIENTED_EDGE('',*,*,#7699,.F.);
#10862=ORIENTED_EDGE('',*,*,#7814,.F.);
#10863=ORIENTED_EDGE('',*,*,#7648,.F.);
#10864=ORIENTED_EDGE('',*,*,#7814,.T.);
#10865=ORIENTED_EDGE('',*,*,#7698,.F.);
#10866=ORIENTED_EDGE('',*,*,#7815,.T.);
#10867=ORIENTED_EDGE('',*,*,#7649,.T.);
#10868=ORIENTED_EDGE('',*,*,#7815,.F.);
#10869=ORIENTED_EDGE('',*,*,#7697,.F.);
#10870=ORIENTED_EDGE('',*,*,#7816,.F.);
#10871=ORIENTED_EDGE('',*,*,#7650,.F.);
#10872=ORIENTED_EDGE('',*,*,#7816,.T.);
#10873=ORIENTED_EDGE('',*,*,#7696,.F.);
#10874=ORIENTED_EDGE('',*,*,#7817,.T.);
#10875=ORIENTED_EDGE('',*,*,#7651,.T.);
#10876=ORIENTED_EDGE('',*,*,#7817,.F.);
#10877=ORIENTED_EDGE('',*,*,#7695,.F.);
#10878=ORIENTED_EDGE('',*,*,#7818,.F.);
#10879=ORIENTED_EDGE('',*,*,#7652,.F.);
#10880=ORIENTED_EDGE('',*,*,#7818,.T.);
#10881=ORIENTED_EDGE('',*,*,#7694,.F.);
#10882=ORIENTED_EDGE('',*,*,#7819,.T.);
#10883=ORIENTED_EDGE('',*,*,#7653,.T.);
#10884=ORIENTED_EDGE('',*,*,#7819,.F.);
#10885=ORIENTED_EDGE('',*,*,#7693,.F.);
#10886=ORIENTED_EDGE('',*,*,#7820,.F.);
#10887=ORIENTED_EDGE('',*,*,#7654,.F.);
#10888=ORIENTED_EDGE('',*,*,#7820,.T.);
#10889=ORIENTED_EDGE('',*,*,#7692,.F.);
#10890=ORIENTED_EDGE('',*,*,#7821,.T.);
#10891=ORIENTED_EDGE('',*,*,#7655,.T.);
#10892=ORIENTED_EDGE('',*,*,#7821,.F.);
#10893=ORIENTED_EDGE('',*,*,#7691,.F.);
#10894=ORIENTED_EDGE('',*,*,#7822,.F.);
#10895=ORIENTED_EDGE('',*,*,#7656,.F.);
#10896=ORIENTED_EDGE('',*,*,#7822,.T.);
#10897=ORIENTED_EDGE('',*,*,#7690,.F.);
#10898=ORIENTED_EDGE('',*,*,#7823,.T.);
#10899=ORIENTED_EDGE('',*,*,#7657,.T.);
#10900=ORIENTED_EDGE('',*,*,#7823,.F.);
#10901=ORIENTED_EDGE('',*,*,#7689,.F.);
#10902=ORIENTED_EDGE('',*,*,#7824,.F.);
#10903=ORIENTED_EDGE('',*,*,#7658,.F.);
#10904=ORIENTED_EDGE('',*,*,#7824,.T.);
#10905=ORIENTED_EDGE('',*,*,#7688,.F.);
#10906=ORIENTED_EDGE('',*,*,#7825,.T.);
#10907=ORIENTED_EDGE('',*,*,#7659,.T.);
#10908=ORIENTED_EDGE('',*,*,#7825,.F.);
#10909=ORIENTED_EDGE('',*,*,#7687,.F.);
#10910=ORIENTED_EDGE('',*,*,#7826,.F.);
#10911=ORIENTED_EDGE('',*,*,#7660,.F.);
#10912=ORIENTED_EDGE('',*,*,#7826,.T.);
#10913=ORIENTED_EDGE('',*,*,#7686,.F.);
#10914=ORIENTED_EDGE('',*,*,#7827,.T.);
#10915=ORIENTED_EDGE('',*,*,#7661,.T.);
#10916=ORIENTED_EDGE('',*,*,#7827,.F.);
#10917=ORIENTED_EDGE('',*,*,#7685,.F.);
#10918=ORIENTED_EDGE('',*,*,#7828,.F.);
#10919=ORIENTED_EDGE('',*,*,#7662,.F.);
#10920=ORIENTED_EDGE('',*,*,#7828,.T.);
#10921=ORIENTED_EDGE('',*,*,#7684,.F.);
#10922=ORIENTED_EDGE('',*,*,#7829,.T.);
#10923=ORIENTED_EDGE('',*,*,#7663,.T.);
#10924=ORIENTED_EDGE('',*,*,#7829,.F.);
#10925=ORIENTED_EDGE('',*,*,#7683,.F.);
#10926=ORIENTED_EDGE('',*,*,#7830,.F.);
#10927=ORIENTED_EDGE('',*,*,#7664,.F.);
#10928=ORIENTED_EDGE('',*,*,#7830,.T.);
#10929=ORIENTED_EDGE('',*,*,#7682,.F.);
#10930=ORIENTED_EDGE('',*,*,#7831,.T.);
#10931=ORIENTED_EDGE('',*,*,#7665,.T.);
#10932=ORIENTED_EDGE('',*,*,#7831,.F.);
#10933=ORIENTED_EDGE('',*,*,#7681,.F.);
#10934=ORIENTED_EDGE('',*,*,#7832,.F.);
#10935=ORIENTED_EDGE('',*,*,#7666,.F.);
#10936=ORIENTED_EDGE('',*,*,#7832,.T.);
#10937=ORIENTED_EDGE('',*,*,#7680,.F.);
#10938=ORIENTED_EDGE('',*,*,#7833,.T.);
#10939=ORIENTED_EDGE('',*,*,#7667,.T.);
#10940=ORIENTED_EDGE('',*,*,#7834,.F.);
#10941=ORIENTED_EDGE('',*,*,#7668,.F.);
#10942=ORIENTED_EDGE('',*,*,#7833,.F.);
#10943=ORIENTED_EDGE('',*,*,#7679,.F.);
#10944=ORIENTED_EDGE('',*,*,#7757,.T.);
#10945=ORIENTED_EDGE('',*,*,#7671,.T.);
#10946=ORIENTED_EDGE('',*,*,#7835,.T.);
#10947=ORIENTED_EDGE('',*,*,#7676,.F.);
#10948=ORIENTED_EDGE('',*,*,#7836,.F.);
#10949=ORIENTED_EDGE('',*,*,#7677,.F.);
#10950=ORIENTED_EDGE('',*,*,#7835,.F.);
#10951=ORIENTED_EDGE('',*,*,#7670,.F.);
#10952=ORIENTED_EDGE('',*,*,#7834,.T.);
#10953=ORIENTED_EDGE('',*,*,#7678,.F.);
#10954=ORIENTED_EDGE('',*,*,#7836,.T.);
#10955=ORIENTED_EDGE('',*,*,#7669,.T.);
#11391=CYLINDRICAL_SURFACE('',#14072,0.125);
#11392=CYLINDRICAL_SURFACE('',#14073,0.125);
#11393=CYLINDRICAL_SURFACE('',#14074,1.);
#11394=CYLINDRICAL_SURFACE('',#14077,0.125);
#11395=CYLINDRICAL_SURFACE('',#14078,0.125);
#11396=CYLINDRICAL_SURFACE('',#14079,0.6);
#11397=CYLINDRICAL_SURFACE('',#14165,1.4);
#11398=CYLINDRICAL_SURFACE('',#14250,1.4);
#11399=CYLINDRICAL_SURFACE('',#14253,0.0555000000000001);
#11400=CYLINDRICAL_SURFACE('',#14254,1.24783954473516);
#11401=CYLINDRICAL_SURFACE('',#14255,0.0555000000000001);
#11402=CYLINDRICAL_SURFACE('',#14256,1.24783954473516);
#11403=CYLINDRICAL_SURFACE('',#14257,0.0555000000000001);
#11404=CYLINDRICAL_SURFACE('',#14258,1.24783954473516);
#11405=CYLINDRICAL_SURFACE('',#14259,0.0555000000000001);
#11406=CYLINDRICAL_SURFACE('',#14260,1.24783954473516);
#11407=CYLINDRICAL_SURFACE('',#14261,0.0555000000000001);
#11408=CYLINDRICAL_SURFACE('',#14262,1.24783954473516);
#11409=CYLINDRICAL_SURFACE('',#14263,0.0555000000000001);
#11410=CYLINDRICAL_SURFACE('',#14264,1.24783954473516);
#11411=CYLINDRICAL_SURFACE('',#14265,0.0555000000000001);
#11412=CYLINDRICAL_SURFACE('',#14266,1.24783954473516);
#11413=CYLINDRICAL_SURFACE('',#14267,0.0555000000000001);
#11414=CYLINDRICAL_SURFACE('',#14268,1.24783954473516);
#11415=CYLINDRICAL_SURFACE('',#14269,0.0555000000000001);
#11416=CYLINDRICAL_SURFACE('',#14270,1.24783954473516);
#11417=CYLINDRICAL_SURFACE('',#14271,0.0555000000000001);
#11418=CYLINDRICAL_SURFACE('',#14272,1.24783954473516);
#11419=CYLINDRICAL_SURFACE('',#14273,0.0555000000000001);
#11420=CYLINDRICAL_SURFACE('',#14274,1.24783954473516);
#11421=CYLINDRICAL_SURFACE('',#14275,0.0555000000000001);
#11422=CYLINDRICAL_SURFACE('',#14276,1.24783954473516);
#11423=CYLINDRICAL_SURFACE('',#14277,0.0555000000000001);
#11424=CYLINDRICAL_SURFACE('',#14278,1.24783954473516);
#11425=CYLINDRICAL_SURFACE('',#14279,0.0555000000000001);
#11426=CYLINDRICAL_SURFACE('',#14280,1.24783954473516);
#11427=CYLINDRICAL_SURFACE('',#14281,0.0555000000000001);
#11428=CYLINDRICAL_SURFACE('',#14282,1.24783954473516);
#11429=CYLINDRICAL_SURFACE('',#14283,0.0555000000000001);
#11430=CYLINDRICAL_SURFACE('',#14284,1.24783954473516);
#11431=CYLINDRICAL_SURFACE('',#14285,0.0555000000000001);
#11432=CYLINDRICAL_SURFACE('',#14286,1.24783954473516);
#11433=CYLINDRICAL_SURFACE('',#14287,0.0555000000000001);
#11434=CYLINDRICAL_SURFACE('',#14288,1.24783954473516);
#11435=CYLINDRICAL_SURFACE('',#14289,0.0555000000000001);
#11436=CYLINDRICAL_SURFACE('',#14290,1.24783954473516);
#11437=CYLINDRICAL_SURFACE('',#14291,0.0555000000000001);
#11438=CYLINDRICAL_SURFACE('',#14292,1.24783954473516);
#11439=CYLINDRICAL_SURFACE('',#14293,0.0555000000000001);
#11440=CYLINDRICAL_SURFACE('',#14294,1.24783954473516);
#11441=CYLINDRICAL_SURFACE('',#14295,0.0555000000000001);
#11442=CYLINDRICAL_SURFACE('',#14296,1.24783954473516);
#11443=CYLINDRICAL_SURFACE('',#14297,0.0555000000000001);
#11444=CYLINDRICAL_SURFACE('',#14298,1.24783954473516);
#11445=CYLINDRICAL_SURFACE('',#14299,0.0555000000000001);
#11446=CYLINDRICAL_SURFACE('',#14300,1.24783954473516);
#11447=CYLINDRICAL_SURFACE('',#14301,0.0555000000000001);
#11448=CYLINDRICAL_SURFACE('',#14302,1.24783954473516);
#11449=CYLINDRICAL_SURFACE('',#14303,0.0555000000000001);
#11450=CYLINDRICAL_SURFACE('',#14304,1.24783954473516);
#11451=CYLINDRICAL_SURFACE('',#14305,0.0555000000000001);
#11452=CYLINDRICAL_SURFACE('',#14306,1.24783954473516);
#11453=CYLINDRICAL_SURFACE('',#14307,0.0555000000000001);
#11454=CYLINDRICAL_SURFACE('',#14308,1.24783954473516);
#11455=CYLINDRICAL_SURFACE('',#14309,0.0555000000000001);
#11456=CYLINDRICAL_SURFACE('',#14310,1.24783954473516);
#11457=CYLINDRICAL_SURFACE('',#14311,0.0555000000000001);
#11458=CYLINDRICAL_SURFACE('',#14312,1.24783954473516);
#11459=CYLINDRICAL_SURFACE('',#14313,0.0555000000000001);
#11460=CYLINDRICAL_SURFACE('',#14314,1.24783954473516);
#11461=CYLINDRICAL_SURFACE('',#14315,0.0555000000000001);
#11462=CYLINDRICAL_SURFACE('',#14316,1.24783954473516);
#11463=CYLINDRICAL_SURFACE('',#14317,0.0555000000000001);
#11464=CYLINDRICAL_SURFACE('',#14318,1.24783954473516);
#11465=CYLINDRICAL_SURFACE('',#14319,0.0555000000000001);
#11466=CYLINDRICAL_SURFACE('',#14320,1.24783954473516);
#11467=CYLINDRICAL_SURFACE('',#14321,0.0555000000000001);
#11468=CYLINDRICAL_SURFACE('',#14322,1.24783954473516);
#11469=CYLINDRICAL_SURFACE('',#14323,0.0555000000000001);
#11470=CYLINDRICAL_SURFACE('',#14324,1.24783954473516);
#11471=CYLINDRICAL_SURFACE('',#14325,0.0555000000000001);
#11472=CYLINDRICAL_SURFACE('',#14326,1.24783954473516);
#11473=CYLINDRICAL_SURFACE('',#14327,0.0555000000000001);
#11474=CYLINDRICAL_SURFACE('',#14328,1.24783954473516);
#11475=CYLINDRICAL_SURFACE('',#14329,0.0555000000000001);
#11476=CYLINDRICAL_SURFACE('',#14330,1.24783954473516);
#11477=CYLINDRICAL_SURFACE('',#14331,0.0555000000000001);
#11478=CYLINDRICAL_SURFACE('',#14332,1.24783954473516);
#12051=ADVANCED_FACE('',(#1910),#11391,.F.);
#12052=ADVANCED_FACE('',(#1911),#11392,.F.);
#12053=ADVANCED_FACE('',(#1912,#1015,#1016,#1017),#11393,.T.);
#12054=ADVANCED_FACE('',(#1913),#11394,.F.);
#12055=ADVANCED_FACE('',(#1914),#11395,.F.);
#12056=ADVANCED_FACE('',(#1915,#1018,#1019,#1020),#11396,.F.);
#12057=ADVANCED_FACE('',(#1916,#1021),#1314,.F.);
#12058=ADVANCED_FACE('',(#1917,#1022),#1315,.T.);
#12059=ADVANCED_FACE('',(#1918),#11397,.T.);
#12060=ADVANCED_FACE('',(#1919,#1023),#1316,.F.);
#12061=ADVANCED_FACE('',(#1920,#1024),#1317,.F.);
#12062=ADVANCED_FACE('',(#1921),#11398,.T.);
#12063=ADVANCED_FACE('',(#1922,#1025),#1318,.T.);
#12064=ADVANCED_FACE('',(#1923),#11399,.F.);
#12065=ADVANCED_FACE('',(#1924),#11400,.T.);
#12066=ADVANCED_FACE('',(#1925),#11401,.F.);
#12067=ADVANCED_FACE('',(#1926),#11402,.T.);
#12068=ADVANCED_FACE('',(#1927),#11403,.F.);
#12069=ADVANCED_FACE('',(#1928),#11404,.T.);
#12070=ADVANCED_FACE('',(#1929),#11405,.F.);
#12071=ADVANCED_FACE('',(#1930),#11406,.T.);
#12072=ADVANCED_FACE('',(#1931),#11407,.F.);
#12073=ADVANCED_FACE('',(#1932),#11408,.T.);
#12074=ADVANCED_FACE('',(#1933),#11409,.F.);
#12075=ADVANCED_FACE('',(#1934),#11410,.T.);
#12076=ADVANCED_FACE('',(#1935),#11411,.F.);
#12077=ADVANCED_FACE('',(#1936),#11412,.T.);
#12078=ADVANCED_FACE('',(#1937),#11413,.F.);
#12079=ADVANCED_FACE('',(#1938),#11414,.T.);
#12080=ADVANCED_FACE('',(#1939),#11415,.F.);
#12081=ADVANCED_FACE('',(#1940),#11416,.T.);
#12082=ADVANCED_FACE('',(#1941),#11417,.F.);
#12083=ADVANCED_FACE('',(#1942),#11418,.T.);
#12084=ADVANCED_FACE('',(#1943),#11419,.F.);
#12085=ADVANCED_FACE('',(#1944),#11420,.T.);
#12086=ADVANCED_FACE('',(#1945),#11421,.F.);
#12087=ADVANCED_FACE('',(#1946),#11422,.T.);
#12088=ADVANCED_FACE('',(#1947),#11423,.F.);
#12089=ADVANCED_FACE('',(#1948),#11424,.T.);
#12090=ADVANCED_FACE('',(#1949),#11425,.F.);
#12091=ADVANCED_FACE('',(#1950),#11426,.T.);
#12092=ADVANCED_FACE('',(#1951),#11427,.F.);
#12093=ADVANCED_FACE('',(#1952),#11428,.T.);
#12094=ADVANCED_FACE('',(#1953),#11429,.F.);
#12095=ADVANCED_FACE('',(#1954),#11430,.T.);
#12096=ADVANCED_FACE('',(#1955),#11431,.F.);
#12097=ADVANCED_FACE('',(#1956),#11432,.T.);
#12098=ADVANCED_FACE('',(#1957),#11433,.F.);
#12099=ADVANCED_FACE('',(#1958),#11434,.T.);
#12100=ADVANCED_FACE('',(#1959),#11435,.F.);
#12101=ADVANCED_FACE('',(#1960),#11436,.T.);
#12102=ADVANCED_FACE('',(#1961),#11437,.F.);
#12103=ADVANCED_FACE('',(#1962),#11438,.T.);
#12104=ADVANCED_FACE('',(#1963),#11439,.F.);
#12105=ADVANCED_FACE('',(#1964),#11440,.T.);
#12106=ADVANCED_FACE('',(#1965),#11441,.F.);
#12107=ADVANCED_FACE('',(#1966),#11442,.T.);
#12108=ADVANCED_FACE('',(#1967),#11443,.F.);
#12109=ADVANCED_FACE('',(#1968),#11444,.T.);
#12110=ADVANCED_FACE('',(#1969),#11445,.F.);
#12111=ADVANCED_FACE('',(#1970),#11446,.T.);
#12112=ADVANCED_FACE('',(#1971),#11447,.F.);
#12113=ADVANCED_FACE('',(#1972),#11448,.T.);
#12114=ADVANCED_FACE('',(#1973),#11449,.F.);
#12115=ADVANCED_FACE('',(#1974),#11450,.T.);
#12116=ADVANCED_FACE('',(#1975),#11451,.F.);
#12117=ADVANCED_FACE('',(#1976),#11452,.T.);
#12118=ADVANCED_FACE('',(#1977),#11453,.F.);
#12119=ADVANCED_FACE('',(#1978),#11454,.T.);
#12120=ADVANCED_FACE('',(#1979),#11455,.F.);
#12121=ADVANCED_FACE('',(#1980),#11456,.T.);
#12122=ADVANCED_FACE('',(#1981),#11457,.F.);
#12123=ADVANCED_FACE('',(#1982),#11458,.T.);
#12124=ADVANCED_FACE('',(#1983),#11459,.F.);
#12125=ADVANCED_FACE('',(#1984),#11460,.T.);
#12126=ADVANCED_FACE('',(#1985),#11461,.F.);
#12127=ADVANCED_FACE('',(#1986),#11462,.T.);
#12128=ADVANCED_FACE('',(#1987),#11463,.F.);
#12129=ADVANCED_FACE('',(#1988),#11464,.T.);
#12130=ADVANCED_FACE('',(#1989),#11465,.F.);
#12131=ADVANCED_FACE('',(#1990),#11466,.T.);
#12132=ADVANCED_FACE('',(#1991),#11467,.F.);
#12133=ADVANCED_FACE('',(#1992),#11468,.T.);
#12134=ADVANCED_FACE('',(#1993),#11469,.F.);
#12135=ADVANCED_FACE('',(#1994),#11470,.T.);
#12136=ADVANCED_FACE('',(#1995),#11471,.F.);
#12137=ADVANCED_FACE('',(#1996),#11472,.T.);
#12138=ADVANCED_FACE('',(#1997),#11473,.F.);
#12139=ADVANCED_FACE('',(#1998),#11474,.T.);
#12140=ADVANCED_FACE('',(#1999),#11475,.F.);
#12141=ADVANCED_FACE('',(#2000),#11476,.T.);
#12142=ADVANCED_FACE('',(#2001),#11477,.F.);
#12143=ADVANCED_FACE('',(#2002),#11478,.T.);
#12264=CLOSED_SHELL('',(#12051,#12052,#12053,#12054,#12055,#12056,#12057,
#12058,#12059,#12060,#12061,#12062,#12063,#12064,#12065,#12066,#12067,#12068,
#12069,#12070,#12071,#12072,#12073,#12074,#12075,#12076,#12077,#12078,#12079,
#12080,#12081,#12082,#12083,#12084,#12085,#12086,#12087,#12088,#12089,#12090,
#12091,#12092,#12093,#12094,#12095,#12096,#12097,#12098,#12099,#12100,#12101,
#12102,#12103,#12104,#12105,#12106,#12107,#12108,#12109,#12110,#12111,#12112,
#12113,#12114,#12115,#12116,#12117,#12118,#12119,#12120,#12121,#12122,#12123,
#12124,#12125,#12126,#12127,#12128,#12129,#12130,#12131,#12132,#12133,#12134,
#12135,#12136,#12137,#12138,#12139,#12140,#12141,#12142,#12143));
#14071=AXIS2_PLACEMENT_3D('',#22245,#17508,#17509);
#14072=AXIS2_PLACEMENT_3D('',#22246,#17510,#17511);
#14073=AXIS2_PLACEMENT_3D('',#22333,#17513,#17514);
#14074=AXIS2_PLACEMENT_3D('',#22414,#17516,#17517);
#14075=AXIS2_PLACEMENT_3D('',#22416,#17518,#17519);
#14076=AXIS2_PLACEMENT_3D('',#22420,#17522,#17523);
#14077=AXIS2_PLACEMENT_3D('',#22503,#17524,#17525);
#14078=AXIS2_PLACEMENT_3D('',#22543,#17527,#17528);
#14079=AXIS2_PLACEMENT_3D('',#22583,#17530,#17531);
#14080=AXIS2_PLACEMENT_3D('',#22585,#17532,#17533);
#14081=AXIS2_PLACEMENT_3D('',#22589,#17536,#17537);
#14082=AXIS2_PLACEMENT_3D('',#22590,#17538,#17539);
#14083=AXIS2_PLACEMENT_3D('',#22591,#17540,#17541);
#14084=AXIS2_PLACEMENT_3D('',#22593,#17542,#17543);
#14085=AXIS2_PLACEMENT_3D('',#22596,#17544,#17545);
#14086=AXIS2_PLACEMENT_3D('',#22598,#17546,#17547);
#14087=AXIS2_PLACEMENT_3D('',#22600,#17548,#17549);
#14088=AXIS2_PLACEMENT_3D('',#22602,#17550,#17551);
#14089=AXIS2_PLACEMENT_3D('',#22604,#17552,#17553);
#14090=AXIS2_PLACEMENT_3D('',#22606,#17554,#17555);
#14091=AXIS2_PLACEMENT_3D('',#22608,#17556,#17557);
#14092=AXIS2_PLACEMENT_3D('',#22610,#17558,#17559);
#14093=AXIS2_PLACEMENT_3D('',#22612,#17560,#17561);
#14094=AXIS2_PLACEMENT_3D('',#22614,#17562,#17563);
#14095=AXIS2_PLACEMENT_3D('',#22616,#17564,#17565);
#14096=AXIS2_PLACEMENT_3D('',#22618,#17566,#17567);
#14097=AXIS2_PLACEMENT_3D('',#22620,#17568,#17569);
#14098=AXIS2_PLACEMENT_3D('',#22622,#17570,#17571);
#14099=AXIS2_PLACEMENT_3D('',#22624,#17572,#17573);
#14100=AXIS2_PLACEMENT_3D('',#22626,#17574,#17575);
#14101=AXIS2_PLACEMENT_3D('',#22628,#17576,#17577);
#14102=AXIS2_PLACEMENT_3D('',#22630,#17578,#17579);
#14103=AXIS2_PLACEMENT_3D('',#22632,#17580,#17581);
#14104=AXIS2_PLACEMENT_3D('',#22634,#17582,#17583);
#14105=AXIS2_PLACEMENT_3D('',#22636,#17584,#17585);
#14106=AXIS2_PLACEMENT_3D('',#22638,#17586,#17587);
#14107=AXIS2_PLACEMENT_3D('',#22640,#17588,#17589);
#14108=AXIS2_PLACEMENT_3D('',#22642,#17590,#17591);
#14109=AXIS2_PLACEMENT_3D('',#22644,#17592,#17593);
#14110=AXIS2_PLACEMENT_3D('',#22646,#17594,#17595);
#14111=AXIS2_PLACEMENT_3D('',#22648,#17596,#17597);
#14112=AXIS2_PLACEMENT_3D('',#22650,#17598,#17599);
#14113=AXIS2_PLACEMENT_3D('',#22652,#17600,#17601);
#14114=AXIS2_PLACEMENT_3D('',#22654,#17602,#17603);
#14115=AXIS2_PLACEMENT_3D('',#22656,#17604,#17605);
#14116=AXIS2_PLACEMENT_3D('',#22658,#17606,#17607);
#14117=AXIS2_PLACEMENT_3D('',#22660,#17608,#17609);
#14118=AXIS2_PLACEMENT_3D('',#22662,#17610,#17611);
#14119=AXIS2_PLACEMENT_3D('',#22664,#17612,#17613);
#14120=AXIS2_PLACEMENT_3D('',#22666,#17614,#17615);
#14121=AXIS2_PLACEMENT_3D('',#22668,#17616,#17617);
#14122=AXIS2_PLACEMENT_3D('',#22670,#17618,#17619);
#14123=AXIS2_PLACEMENT_3D('',#22672,#17620,#17621);
#14124=AXIS2_PLACEMENT_3D('',#22674,#17622,#17623);
#14125=AXIS2_PLACEMENT_3D('',#22676,#17624,#17625);
#14126=AXIS2_PLACEMENT_3D('',#22678,#17626,#17627);
#14127=AXIS2_PLACEMENT_3D('',#22680,#17628,#17629);
#14128=AXIS2_PLACEMENT_3D('',#22682,#17630,#17631);
#14129=AXIS2_PLACEMENT_3D('',#22684,#17632,#17633);
#14130=AXIS2_PLACEMENT_3D('',#22686,#17634,#17635);
#14131=AXIS2_PLACEMENT_3D('',#22688,#17636,#17637);
#14132=AXIS2_PLACEMENT_3D('',#22690,#17638,#17639);
#14133=AXIS2_PLACEMENT_3D('',#22692,#17640,#17641);
#14134=AXIS2_PLACEMENT_3D('',#22694,#17642,#17643);
#14135=AXIS2_PLACEMENT_3D('',#22696,#17644,#17645);
#14136=AXIS2_PLACEMENT_3D('',#22698,#17646,#17647);
#14137=AXIS2_PLACEMENT_3D('',#22700,#17648,#17649);
#14138=AXIS2_PLACEMENT_3D('',#22702,#17650,#17651);
#14139=AXIS2_PLACEMENT_3D('',#22704,#17652,#17653);
#14140=AXIS2_PLACEMENT_3D('',#22706,#17654,#17655);
#14141=AXIS2_PLACEMENT_3D('',#22708,#17656,#17657);
#14142=AXIS2_PLACEMENT_3D('',#22710,#17658,#17659);
#14143=AXIS2_PLACEMENT_3D('',#22712,#17660,#17661);
#14144=AXIS2_PLACEMENT_3D('',#22714,#17662,#17663);
#14145=AXIS2_PLACEMENT_3D('',#22716,#17664,#17665);
#14146=AXIS2_PLACEMENT_3D('',#22718,#17666,#17667);
#14147=AXIS2_PLACEMENT_3D('',#22720,#17668,#17669);
#14148=AXIS2_PLACEMENT_3D('',#22722,#17670,#17671);
#14149=AXIS2_PLACEMENT_3D('',#22724,#17672,#17673);
#14150=AXIS2_PLACEMENT_3D('',#22726,#17674,#17675);
#14151=AXIS2_PLACEMENT_3D('',#22728,#17676,#17677);
#14152=AXIS2_PLACEMENT_3D('',#22730,#17678,#17679);
#14153=AXIS2_PLACEMENT_3D('',#22732,#17680,#17681);
#14154=AXIS2_PLACEMENT_3D('',#22734,#17682,#17683);
#14155=AXIS2_PLACEMENT_3D('',#22736,#17684,#17685);
#14156=AXIS2_PLACEMENT_3D('',#22738,#17686,#17687);
#14157=AXIS2_PLACEMENT_3D('',#22740,#17688,#17689);
#14158=AXIS2_PLACEMENT_3D('',#22742,#17690,#17691);
#14159=AXIS2_PLACEMENT_3D('',#22744,#17692,#17693);
#14160=AXIS2_PLACEMENT_3D('',#22746,#17694,#17695);
#14161=AXIS2_PLACEMENT_3D('',#22748,#17696,#17697);
#14162=AXIS2_PLACEMENT_3D('',#22750,#17698,#17699);
#14163=AXIS2_PLACEMENT_3D('',#22752,#17700,#17701);
#14164=AXIS2_PLACEMENT_3D('',#22753,#17702,#17703);
#14165=AXIS2_PLACEMENT_3D('',#22754,#17704,#17705);
#14166=AXIS2_PLACEMENT_3D('',#22756,#17706,#17707);
#14167=AXIS2_PLACEMENT_3D('',#22758,#17709,#17710);
#14168=AXIS2_PLACEMENT_3D('',#22759,#17711,#17712);
#14169=AXIS2_PLACEMENT_3D('',#22761,#17713,#17714);
#14170=AXIS2_PLACEMENT_3D('',#22764,#17715,#17716);
#14171=AXIS2_PLACEMENT_3D('',#22766,#17717,#17718);
#14172=AXIS2_PLACEMENT_3D('',#22768,#17719,#17720);
#14173=AXIS2_PLACEMENT_3D('',#22770,#17721,#17722);
#14174=AXIS2_PLACEMENT_3D('',#22772,#17723,#17724);
#14175=AXIS2_PLACEMENT_3D('',#22774,#17725,#17726);
#14176=AXIS2_PLACEMENT_3D('',#22776,#17727,#17728);
#14177=AXIS2_PLACEMENT_3D('',#22778,#17729,#17730);
#14178=AXIS2_PLACEMENT_3D('',#22780,#17731,#17732);
#14179=AXIS2_PLACEMENT_3D('',#22782,#17733,#17734);
#14180=AXIS2_PLACEMENT_3D('',#22784,#17735,#17736);
#14181=AXIS2_PLACEMENT_3D('',#22786,#17737,#17738);
#14182=AXIS2_PLACEMENT_3D('',#22788,#17739,#17740);
#14183=AXIS2_PLACEMENT_3D('',#22790,#17741,#17742);
#14184=AXIS2_PLACEMENT_3D('',#22792,#17743,#17744);
#14185=AXIS2_PLACEMENT_3D('',#22794,#17745,#17746);
#14186=AXIS2_PLACEMENT_3D('',#22796,#17747,#17748);
#14187=AXIS2_PLACEMENT_3D('',#22798,#17749,#17750);
#14188=AXIS2_PLACEMENT_3D('',#22800,#17751,#17752);
#14189=AXIS2_PLACEMENT_3D('',#22802,#17753,#17754);
#14190=AXIS2_PLACEMENT_3D('',#22804,#17755,#17756);
#14191=AXIS2_PLACEMENT_3D('',#22806,#17757,#17758);
#14192=AXIS2_PLACEMENT_3D('',#22808,#17759,#17760);
#14193=AXIS2_PLACEMENT_3D('',#22810,#17761,#17762);
#14194=AXIS2_PLACEMENT_3D('',#22812,#17763,#17764);
#14195=AXIS2_PLACEMENT_3D('',#22814,#17765,#17766);
#14196=AXIS2_PLACEMENT_3D('',#22816,#17767,#17768);
#14197=AXIS2_PLACEMENT_3D('',#22818,#17769,#17770);
#14198=AXIS2_PLACEMENT_3D('',#22820,#17771,#17772);
#14199=AXIS2_PLACEMENT_3D('',#22822,#17773,#17774);
#14200=AXIS2_PLACEMENT_3D('',#22824,#17775,#17776);
#14201=AXIS2_PLACEMENT_3D('',#22826,#17777,#17778);
#14202=AXIS2_PLACEMENT_3D('',#22828,#17779,#17780);
#14203=AXIS2_PLACEMENT_3D('',#22830,#17781,#17782);
#14204=AXIS2_PLACEMENT_3D('',#22832,#17783,#17784);
#14205=AXIS2_PLACEMENT_3D('',#22834,#17785,#17786);
#14206=AXIS2_PLACEMENT_3D('',#22836,#17787,#17788);
#14207=AXIS2_PLACEMENT_3D('',#22838,#17789,#17790);
#14208=AXIS2_PLACEMENT_3D('',#22840,#17791,#17792);
#14209=AXIS2_PLACEMENT_3D('',#22842,#17793,#17794);
#14210=AXIS2_PLACEMENT_3D('',#22844,#17795,#17796);
#14211=AXIS2_PLACEMENT_3D('',#22846,#17797,#17798);
#14212=AXIS2_PLACEMENT_3D('',#22848,#17799,#17800);
#14213=AXIS2_PLACEMENT_3D('',#22850,#17801,#17802);
#14214=AXIS2_PLACEMENT_3D('',#22852,#17803,#17804);
#14215=AXIS2_PLACEMENT_3D('',#22854,#17805,#17806);
#14216=AXIS2_PLACEMENT_3D('',#22856,#17807,#17808);
#14217=AXIS2_PLACEMENT_3D('',#22858,#17809,#17810);
#14218=AXIS2_PLACEMENT_3D('',#22860,#17811,#17812);
#14219=AXIS2_PLACEMENT_3D('',#22862,#17813,#17814);
#14220=AXIS2_PLACEMENT_3D('',#22864,#17815,#17816);
#14221=AXIS2_PLACEMENT_3D('',#22866,#17817,#17818);
#14222=AXIS2_PLACEMENT_3D('',#22868,#17819,#17820);
#14223=AXIS2_PLACEMENT_3D('',#22870,#17821,#17822);
#14224=AXIS2_PLACEMENT_3D('',#22872,#17823,#17824);
#14225=AXIS2_PLACEMENT_3D('',#22874,#17825,#17826);
#14226=AXIS2_PLACEMENT_3D('',#22876,#17827,#17828);
#14227=AXIS2_PLACEMENT_3D('',#22878,#17829,#17830);
#14228=AXIS2_PLACEMENT_3D('',#22880,#17831,#17832);
#14229=AXIS2_PLACEMENT_3D('',#22882,#17833,#17834);
#14230=AXIS2_PLACEMENT_3D('',#22884,#17835,#17836);
#14231=AXIS2_PLACEMENT_3D('',#22886,#17837,#17838);
#14232=AXIS2_PLACEMENT_3D('',#22888,#17839,#17840);
#14233=AXIS2_PLACEMENT_3D('',#22890,#17841,#17842);
#14234=AXIS2_PLACEMENT_3D('',#22892,#17843,#17844);
#14235=AXIS2_PLACEMENT_3D('',#22894,#17845,#17846);
#14236=AXIS2_PLACEMENT_3D('',#22896,#17847,#17848);
#14237=AXIS2_PLACEMENT_3D('',#22898,#17849,#17850);
#14238=AXIS2_PLACEMENT_3D('',#22900,#17851,#17852);
#14239=AXIS2_PLACEMENT_3D('',#22902,#17853,#17854);
#14240=AXIS2_PLACEMENT_3D('',#22904,#17855,#17856);
#14241=AXIS2_PLACEMENT_3D('',#22906,#17857,#17858);
#14242=AXIS2_PLACEMENT_3D('',#22908,#17859,#17860);
#14243=AXIS2_PLACEMENT_3D('',#22910,#17861,#17862);
#14244=AXIS2_PLACEMENT_3D('',#22912,#17863,#17864);
#14245=AXIS2_PLACEMENT_3D('',#22914,#17865,#17866);
#14246=AXIS2_PLACEMENT_3D('',#22916,#17867,#17868);
#14247=AXIS2_PLACEMENT_3D('',#22918,#17869,#17870);
#14248=AXIS2_PLACEMENT_3D('',#22920,#17871,#17872);
#14249=AXIS2_PLACEMENT_3D('',#22921,#17873,#17874);
#14250=AXIS2_PLACEMENT_3D('',#22922,#17875,#17876);
#14251=AXIS2_PLACEMENT_3D('',#22924,#17877,#17878);
#14252=AXIS2_PLACEMENT_3D('',#22926,#17880,#17881);
#14253=AXIS2_PLACEMENT_3D('',#22927,#17882,#17883);
#14254=AXIS2_PLACEMENT_3D('',#22930,#17886,#17887);
#14255=AXIS2_PLACEMENT_3D('',#22932,#17889,#17890);
#14256=AXIS2_PLACEMENT_3D('',#22934,#17892,#17893);
#14257=AXIS2_PLACEMENT_3D('',#22936,#17895,#17896);
#14258=AXIS2_PLACEMENT_3D('',#22938,#17898,#17899);
#14259=AXIS2_PLACEMENT_3D('',#22940,#17901,#17902);
#14260=AXIS2_PLACEMENT_3D('',#22942,#17904,#17905);
#14261=AXIS2_PLACEMENT_3D('',#22944,#17907,#17908);
#14262=AXIS2_PLACEMENT_3D('',#22946,#17910,#17911);
#14263=AXIS2_PLACEMENT_3D('',#22948,#17913,#17914);
#14264=AXIS2_PLACEMENT_3D('',#22950,#17916,#17917);
#14265=AXIS2_PLACEMENT_3D('',#22952,#17919,#17920);
#14266=AXIS2_PLACEMENT_3D('',#22954,#17922,#17923);
#14267=AXIS2_PLACEMENT_3D('',#22956,#17925,#17926);
#14268=AXIS2_PLACEMENT_3D('',#22958,#17928,#17929);
#14269=AXIS2_PLACEMENT_3D('',#22960,#17931,#17932);
#14270=AXIS2_PLACEMENT_3D('',#22962,#17934,#17935);
#14271=AXIS2_PLACEMENT_3D('',#22964,#17937,#17938);
#14272=AXIS2_PLACEMENT_3D('',#22966,#17940,#17941);
#14273=AXIS2_PLACEMENT_3D('',#22968,#17943,#17944);
#14274=AXIS2_PLACEMENT_3D('',#22970,#17946,#17947);
#14275=AXIS2_PLACEMENT_3D('',#22972,#17949,#17950);
#14276=AXIS2_PLACEMENT_3D('',#22974,#17952,#17953);
#14277=AXIS2_PLACEMENT_3D('',#22976,#17955,#17956);
#14278=AXIS2_PLACEMENT_3D('',#22978,#17958,#17959);
#14279=AXIS2_PLACEMENT_3D('',#22980,#17961,#17962);
#14280=AXIS2_PLACEMENT_3D('',#22982,#17964,#17965);
#14281=AXIS2_PLACEMENT_3D('',#22984,#17967,#17968);
#14282=AXIS2_PLACEMENT_3D('',#22986,#17970,#17971);
#14283=AXIS2_PLACEMENT_3D('',#22988,#17973,#17974);
#14284=AXIS2_PLACEMENT_3D('',#22990,#17976,#17977);
#14285=AXIS2_PLACEMENT_3D('',#22992,#17979,#17980);
#14286=AXIS2_PLACEMENT_3D('',#22994,#17982,#17983);
#14287=AXIS2_PLACEMENT_3D('',#22996,#17985,#17986);
#14288=AXIS2_PLACEMENT_3D('',#22998,#17988,#17989);
#14289=AXIS2_PLACEMENT_3D('',#23000,#17991,#17992);
#14290=AXIS2_PLACEMENT_3D('',#23002,#17994,#17995);
#14291=AXIS2_PLACEMENT_3D('',#23004,#17997,#17998);
#14292=AXIS2_PLACEMENT_3D('',#23006,#18000,#18001);
#14293=AXIS2_PLACEMENT_3D('',#23008,#18003,#18004);
#14294=AXIS2_PLACEMENT_3D('',#23010,#18006,#18007);
#14295=AXIS2_PLACEMENT_3D('',#23012,#18009,#18010);
#14296=AXIS2_PLACEMENT_3D('',#23014,#18012,#18013);
#14297=AXIS2_PLACEMENT_3D('',#23016,#18015,#18016);
#14298=AXIS2_PLACEMENT_3D('',#23018,#18018,#18019);
#14299=AXIS2_PLACEMENT_3D('',#23020,#18021,#18022);
#14300=AXIS2_PLACEMENT_3D('',#23022,#18024,#18025);
#14301=AXIS2_PLACEMENT_3D('',#23024,#18027,#18028);
#14302=AXIS2_PLACEMENT_3D('',#23026,#18030,#18031);
#14303=AXIS2_PLACEMENT_3D('',#23028,#18033,#18034);
#14304=AXIS2_PLACEMENT_3D('',#23030,#18036,#18037);
#14305=AXIS2_PLACEMENT_3D('',#23032,#18039,#18040);
#14306=AXIS2_PLACEMENT_3D('',#23034,#18042,#18043);
#14307=AXIS2_PLACEMENT_3D('',#23036,#18045,#18046);
#14308=AXIS2_PLACEMENT_3D('',#23038,#18048,#18049);
#14309=AXIS2_PLACEMENT_3D('',#23040,#18051,#18052);
#14310=AXIS2_PLACEMENT_3D('',#23042,#18054,#18055);
#14311=AXIS2_PLACEMENT_3D('',#23044,#18057,#18058);
#14312=AXIS2_PLACEMENT_3D('',#23046,#18060,#18061);
#14313=AXIS2_PLACEMENT_3D('',#23048,#18063,#18064);
#14314=AXIS2_PLACEMENT_3D('',#23050,#18066,#18067);
#14315=AXIS2_PLACEMENT_3D('',#23052,#18069,#18070);
#14316=AXIS2_PLACEMENT_3D('',#23054,#18072,#18073);
#14317=AXIS2_PLACEMENT_3D('',#23056,#18075,#18076);
#14318=AXIS2_PLACEMENT_3D('',#23058,#18078,#18079);
#14319=AXIS2_PLACEMENT_3D('',#23060,#18081,#18082);
#14320=AXIS2_PLACEMENT_3D('',#23062,#18084,#18085);
#14321=AXIS2_PLACEMENT_3D('',#23064,#18087,#18088);
#14322=AXIS2_PLACEMENT_3D('',#23066,#18090,#18091);
#14323=AXIS2_PLACEMENT_3D('',#23068,#18093,#18094);
#14324=AXIS2_PLACEMENT_3D('',#23070,#18096,#18097);
#14325=AXIS2_PLACEMENT_3D('',#23072,#18099,#18100);
#14326=AXIS2_PLACEMENT_3D('',#23074,#18102,#18103);
#14327=AXIS2_PLACEMENT_3D('',#23076,#18105,#18106);
#14328=AXIS2_PLACEMENT_3D('',#23078,#18108,#18109);
#14329=AXIS2_PLACEMENT_3D('',#23080,#18111,#18112);
#14330=AXIS2_PLACEMENT_3D('',#23082,#18114,#18115);
#14331=AXIS2_PLACEMENT_3D('',#23084,#18117,#18118);
#14332=AXIS2_PLACEMENT_3D('',#23086,#18120,#18121);
#17508=DIRECTION('axis',(0.,0.,1.));
#17509=DIRECTION('refdir',(1.,0.,0.));
#17510=DIRECTION('center_axis',(1.,0.,6.12323399573677E-17));
#17511=DIRECTION('ref_axis',(6.12323399573677E-17,0.,-1.));
#17512=DIRECTION('',(1.,0.,6.12323399573677E-17));
#17513=DIRECTION('center_axis',(1.,0.,6.12323399573677E-17));
#17514=DIRECTION('ref_axis',(6.12323399573677E-17,0.,-1.));
#17515=DIRECTION('',(1.,0.,6.12323399573677E-17));
#17516=DIRECTION('center_axis',(0.,-1.,0.));
#17517=DIRECTION('ref_axis',(1.,0.,0.));
#17518=DIRECTION('center_axis',(0.,-1.,0.));
#17519=DIRECTION('ref_axis',(1.,0.,0.));
#17520=DIRECTION('',(0.,1.,0.));
#17521=DIRECTION('',(0.,1.,0.));
#17522=DIRECTION('center_axis',(0.,1.,0.));
#17523=DIRECTION('ref_axis',(1.,0.,0.));
#17524=DIRECTION('center_axis',(0.,0.,1.));
#17525=DIRECTION('ref_axis',(1.,0.,0.));
#17526=DIRECTION('',(0.,0.,1.));
#17527=DIRECTION('center_axis',(0.,0.,1.));
#17528=DIRECTION('ref_axis',(1.,0.,0.));
#17529=DIRECTION('',(0.,0.,1.));
#17530=DIRECTION('center_axis',(0.,1.,0.));
#17531=DIRECTION('ref_axis',(1.,0.,0.));
#17532=DIRECTION('center_axis',(0.,1.,0.));
#17533=DIRECTION('ref_axis',(1.,0.,0.));
#17534=DIRECTION('',(0.,1.,0.));
#17535=DIRECTION('',(0.,1.,0.));
#17536=DIRECTION('center_axis',(0.,-1.,0.));
#17537=DIRECTION('ref_axis',(1.,0.,0.));
#17538=DIRECTION('center_axis',(0.,1.,0.));
#17539=DIRECTION('ref_axis',(1.,0.,0.));
#17540=DIRECTION('center_axis',(0.,1.,0.));
#17541=DIRECTION('ref_axis',(1.,0.,0.));
#17542=DIRECTION('center_axis',(0.,1.,0.));
#17543=DIRECTION('ref_axis',(1.,0.,0.));
#17544=DIRECTION('center_axis',(0.,1.,0.));
#17545=DIRECTION('ref_axis',(0.987688340595138,0.,0.156434465040231));
#17546=DIRECTION('center_axis',(0.,1.,0.));
#17547=DIRECTION('ref_axis',(1.,0.,0.));
#17548=DIRECTION('center_axis',(0.,1.,0.));
#17549=DIRECTION('ref_axis',(0.951056516295154,0.,0.309016994374948));
#17550=DIRECTION('center_axis',(0.,1.,0.));
#17551=DIRECTION('ref_axis',(1.,0.,0.));
#17552=DIRECTION('center_axis',(0.,1.,0.));
#17553=DIRECTION('ref_axis',(0.891006524188368,0.,0.453990499739547));
#17554=DIRECTION('center_axis',(0.,1.,0.));
#17555=DIRECTION('ref_axis',(1.,0.,0.));
#17556=DIRECTION('center_axis',(0.,1.,0.));
#17557=DIRECTION('ref_axis',(0.809016994374947,0.,0.587785252292473));
#17558=DIRECTION('center_axis',(0.,1.,0.));
#17559=DIRECTION('ref_axis',(1.,0.,0.));
#17560=DIRECTION('center_axis',(0.,1.,0.));
#17561=DIRECTION('ref_axis',(0.707106781186547,0.,0.707106781186548));
#17562=DIRECTION('center_axis',(0.,1.,0.));
#17563=DIRECTION('ref_axis',(1.,0.,0.));
#17564=DIRECTION('center_axis',(0.,1.,0.));
#17565=DIRECTION('ref_axis',(0.587785252292473,0.,0.809016994374948));
#17566=DIRECTION('center_axis',(0.,1.,0.));
#17567=DIRECTION('ref_axis',(1.,0.,0.));
#17568=DIRECTION('center_axis',(0.,1.,0.));
#17569=DIRECTION('ref_axis',(0.453990499739547,0.,0.891006524188368));
#17570=DIRECTION('center_axis',(0.,1.,0.));
#17571=DIRECTION('ref_axis',(1.,0.,0.));
#17572=DIRECTION('center_axis',(0.,1.,0.));
#17573=DIRECTION('ref_axis',(0.309016994374947,0.,0.951056516295154));
#17574=DIRECTION('center_axis',(0.,1.,0.));
#17575=DIRECTION('ref_axis',(1.,0.,0.));
#17576=DIRECTION('center_axis',(0.,1.,0.));
#17577=DIRECTION('ref_axis',(0.156434465040231,0.,0.987688340595138));
#17578=DIRECTION('center_axis',(0.,1.,0.));
#17579=DIRECTION('ref_axis',(1.,0.,0.));
#17580=DIRECTION('center_axis',(0.,1.,0.));
#17581=DIRECTION('ref_axis',(-1.83697019872103E-16,0.,1.));
#17582=DIRECTION('center_axis',(0.,1.,0.));
#17583=DIRECTION('ref_axis',(1.,0.,0.));
#17584=DIRECTION('center_axis',(0.,1.,0.));
#17585=DIRECTION('ref_axis',(-0.156434465040231,0.,0.987688340595138));
#17586=DIRECTION('center_axis',(0.,1.,0.));
#17587=DIRECTION('ref_axis',(1.,0.,0.));
#17588=DIRECTION('center_axis',(0.,1.,0.));
#17589=DIRECTION('ref_axis',(-0.309016994374948,0.,0.951056516295154));
#17590=DIRECTION('center_axis',(0.,1.,0.));
#17591=DIRECTION('ref_axis',(1.,0.,0.));
#17592=DIRECTION('center_axis',(0.,1.,0.));
#17593=DIRECTION('ref_axis',(-0.453990499739547,0.,0.891006524188368));
#17594=DIRECTION('center_axis',(0.,1.,0.));
#17595=DIRECTION('ref_axis',(1.,0.,0.));
#17596=DIRECTION('center_axis',(0.,1.,0.));
#17597=DIRECTION('ref_axis',(-0.587785252292473,0.,0.809016994374947));
#17598=DIRECTION('center_axis',(0.,1.,0.));
#17599=DIRECTION('ref_axis',(1.,0.,0.));
#17600=DIRECTION('center_axis',(0.,1.,0.));
#17601=DIRECTION('ref_axis',(-0.707106781186548,0.,0.707106781186547));
#17602=DIRECTION('center_axis',(0.,1.,0.));
#17603=DIRECTION('ref_axis',(1.,0.,0.));
#17604=DIRECTION('center_axis',(0.,1.,0.));
#17605=DIRECTION('ref_axis',(-0.809016994374947,0.,0.587785252292473));
#17606=DIRECTION('center_axis',(0.,1.,0.));
#17607=DIRECTION('ref_axis',(1.,0.,0.));
#17608=DIRECTION('center_axis',(0.,1.,0.));
#17609=DIRECTION('ref_axis',(-0.891006524188368,0.,0.453990499739547));
#17610=DIRECTION('center_axis',(0.,1.,0.));
#17611=DIRECTION('ref_axis',(1.,0.,0.));
#17612=DIRECTION('center_axis',(0.,1.,0.));
#17613=DIRECTION('ref_axis',(-0.951056516295154,0.,0.309016994374947));
#17614=DIRECTION('center_axis',(0.,1.,0.));
#17615=DIRECTION('ref_axis',(1.,0.,0.));
#17616=DIRECTION('center_axis',(0.,1.,0.));
#17617=DIRECTION('ref_axis',(-0.987688340595138,0.,0.156434465040231));
#17618=DIRECTION('center_axis',(0.,1.,0.));
#17619=DIRECTION('ref_axis',(1.,0.,0.));
#17620=DIRECTION('center_axis',(0.,1.,0.));
#17621=DIRECTION('ref_axis',(-1.,0.,-1.22464679914735E-16));
#17622=DIRECTION('center_axis',(0.,1.,0.));
#17623=DIRECTION('ref_axis',(1.,0.,0.));
#17624=DIRECTION('center_axis',(0.,1.,0.));
#17625=DIRECTION('ref_axis',(-0.987688340595138,0.,-0.156434465040231));
#17626=DIRECTION('center_axis',(0.,1.,0.));
#17627=DIRECTION('ref_axis',(1.,0.,0.));
#17628=DIRECTION('center_axis',(0.,1.,0.));
#17629=DIRECTION('ref_axis',(-0.951056516295154,0.,-0.309016994374948));
#17630=DIRECTION('center_axis',(0.,1.,0.));
#17631=DIRECTION('ref_axis',(1.,0.,0.));
#17632=DIRECTION('center_axis',(0.,1.,0.));
#17633=DIRECTION('ref_axis',(-0.891006524188368,0.,-0.453990499739547));
#17634=DIRECTION('center_axis',(0.,1.,0.));
#17635=DIRECTION('ref_axis',(1.,0.,0.));
#17636=DIRECTION('center_axis',(0.,1.,0.));
#17637=DIRECTION('ref_axis',(-0.809016994374947,0.,-0.587785252292473));
#17638=DIRECTION('center_axis',(0.,1.,0.));
#17639=DIRECTION('ref_axis',(1.,0.,0.));
#17640=DIRECTION('center_axis',(0.,1.,0.));
#17641=DIRECTION('ref_axis',(-0.707106781186547,0.,-0.707106781186548));
#17642=DIRECTION('center_axis',(0.,1.,0.));
#17643=DIRECTION('ref_axis',(1.,0.,0.));
#17644=DIRECTION('center_axis',(0.,1.,0.));
#17645=DIRECTION('ref_axis',(-0.587785252292473,0.,-0.809016994374947));
#17646=DIRECTION('center_axis',(0.,1.,0.));
#17647=DIRECTION('ref_axis',(1.,0.,0.));
#17648=DIRECTION('center_axis',(0.,1.,0.));
#17649=DIRECTION('ref_axis',(-0.453990499739547,0.,-0.891006524188368));
#17650=DIRECTION('center_axis',(0.,1.,0.));
#17651=DIRECTION('ref_axis',(1.,0.,0.));
#17652=DIRECTION('center_axis',(0.,1.,0.));
#17653=DIRECTION('ref_axis',(-0.309016994374947,0.,-0.951056516295154));
#17654=DIRECTION('center_axis',(0.,1.,0.));
#17655=DIRECTION('ref_axis',(1.,0.,0.));
#17656=DIRECTION('center_axis',(0.,1.,0.));
#17657=DIRECTION('ref_axis',(-0.156434465040231,0.,-0.987688340595138));
#17658=DIRECTION('center_axis',(0.,1.,0.));
#17659=DIRECTION('ref_axis',(1.,0.,0.));
#17660=DIRECTION('center_axis',(0.,1.,0.));
#17661=DIRECTION('ref_axis',(6.12323399573677E-17,0.,-1.));
#17662=DIRECTION('center_axis',(0.,1.,0.));
#17663=DIRECTION('ref_axis',(1.,0.,0.));
#17664=DIRECTION('center_axis',(0.,1.,0.));
#17665=DIRECTION('ref_axis',(0.156434465040231,0.,-0.987688340595138));
#17666=DIRECTION('center_axis',(0.,1.,0.));
#17667=DIRECTION('ref_axis',(1.,0.,0.));
#17668=DIRECTION('center_axis',(0.,1.,0.));
#17669=DIRECTION('ref_axis',(0.309016994374948,0.,-0.951056516295154));
#17670=DIRECTION('center_axis',(0.,1.,0.));
#17671=DIRECTION('ref_axis',(1.,0.,0.));
#17672=DIRECTION('center_axis',(0.,1.,0.));
#17673=DIRECTION('ref_axis',(0.453990499739547,0.,-0.891006524188368));
#17674=DIRECTION('center_axis',(0.,1.,0.));
#17675=DIRECTION('ref_axis',(1.,0.,0.));
#17676=DIRECTION('center_axis',(0.,1.,0.));
#17677=DIRECTION('ref_axis',(0.587785252292473,0.,-0.809016994374947));
#17678=DIRECTION('center_axis',(0.,1.,0.));
#17679=DIRECTION('ref_axis',(1.,0.,0.));
#17680=DIRECTION('center_axis',(0.,1.,0.));
#17681=DIRECTION('ref_axis',(0.707106781186548,0.,-0.707106781186547));
#17682=DIRECTION('center_axis',(0.,1.,0.));
#17683=DIRECTION('ref_axis',(1.,0.,0.));
#17684=DIRECTION('center_axis',(0.,1.,0.));
#17685=DIRECTION('ref_axis',(0.809016994374947,0.,-0.587785252292473));
#17686=DIRECTION('center_axis',(0.,1.,0.));
#17687=DIRECTION('ref_axis',(1.,0.,0.));
#17688=DIRECTION('center_axis',(0.,1.,0.));
#17689=DIRECTION('ref_axis',(0.891006524188368,0.,-0.453990499739547));
#17690=DIRECTION('center_axis',(0.,1.,0.));
#17691=DIRECTION('ref_axis',(1.,0.,0.));
#17692=DIRECTION('center_axis',(0.,1.,0.));
#17693=DIRECTION('ref_axis',(0.951056516295154,0.,-0.309016994374947));
#17694=DIRECTION('center_axis',(0.,1.,0.));
#17695=DIRECTION('ref_axis',(1.,0.,0.));
#17696=DIRECTION('center_axis',(0.,1.,0.));
#17697=DIRECTION('ref_axis',(0.987688340595138,0.,-0.156434465040231));
#17698=DIRECTION('center_axis',(0.,1.,0.));
#17699=DIRECTION('ref_axis',(1.,0.,0.));
#17700=DIRECTION('center_axis',(0.,1.,0.));
#17701=DIRECTION('ref_axis',(1.,0.,0.));
#17702=DIRECTION('center_axis',(0.,1.,0.));
#17703=DIRECTION('ref_axis',(1.,0.,0.));
#17704=DIRECTION('center_axis',(0.,-1.,0.));
#17705=DIRECTION('ref_axis',(1.,0.,0.));
#17706=DIRECTION('center_axis',(0.,-1.,0.));
#17707=DIRECTION('ref_axis',(1.,0.,0.));
#17708=DIRECTION('',(0.,1.,0.));
#17709=DIRECTION('center_axis',(0.,1.,0.));
#17710=DIRECTION('ref_axis',(1.,0.,0.));
#17711=DIRECTION('center_axis',(0.,1.,0.));
#17712=DIRECTION('ref_axis',(1.,0.,0.));
#17713=DIRECTION('center_axis',(0.,1.,0.));
#17714=DIRECTION('ref_axis',(1.,0.,0.));
#17715=DIRECTION('center_axis',(0.,-1.,0.));
#17716=DIRECTION('ref_axis',(0.987688340595138,0.,0.156434465040231));
#17717=DIRECTION('center_axis',(0.,1.,0.));
#17718=DIRECTION('ref_axis',(1.,0.,0.));
#17719=DIRECTION('center_axis',(0.,-1.,0.));
#17720=DIRECTION('ref_axis',(1.,0.,0.));
#17721=DIRECTION('center_axis',(0.,1.,0.));
#17722=DIRECTION('ref_axis',(1.,0.,0.));
#17723=DIRECTION('center_axis',(0.,-1.,0.));
#17724=DIRECTION('ref_axis',(0.987688340595138,0.,-0.156434465040231));
#17725=DIRECTION('center_axis',(0.,1.,0.));
#17726=DIRECTION('ref_axis',(1.,0.,0.));
#17727=DIRECTION('center_axis',(0.,-1.,0.));
#17728=DIRECTION('ref_axis',(0.951056516295154,0.,-0.309016994374947));
#17729=DIRECTION('center_axis',(0.,1.,0.));
#17730=DIRECTION('ref_axis',(1.,0.,0.));
#17731=DIRECTION('center_axis',(0.,-1.,0.));
#17732=DIRECTION('ref_axis',(0.891006524188368,0.,-0.453990499739547));
#17733=DIRECTION('center_axis',(0.,1.,0.));
#17734=DIRECTION('ref_axis',(1.,0.,0.));
#17735=DIRECTION('center_axis',(0.,-1.,0.));
#17736=DIRECTION('ref_axis',(0.809016994374947,0.,-0.587785252292473));
#17737=DIRECTION('center_axis',(0.,1.,0.));
#17738=DIRECTION('ref_axis',(1.,0.,0.));
#17739=DIRECTION('center_axis',(0.,-1.,0.));
#17740=DIRECTION('ref_axis',(0.707106781186548,0.,-0.707106781186547));
#17741=DIRECTION('center_axis',(0.,1.,0.));
#17742=DIRECTION('ref_axis',(1.,0.,0.));
#17743=DIRECTION('center_axis',(0.,-1.,0.));
#17744=DIRECTION('ref_axis',(0.587785252292473,0.,-0.809016994374947));
#17745=DIRECTION('center_axis',(0.,1.,0.));
#17746=DIRECTION('ref_axis',(1.,0.,0.));
#17747=DIRECTION('center_axis',(0.,-1.,0.));
#17748=DIRECTION('ref_axis',(0.453990499739547,0.,-0.891006524188368));
#17749=DIRECTION('center_axis',(0.,1.,0.));
#17750=DIRECTION('ref_axis',(1.,0.,0.));
#17751=DIRECTION('center_axis',(0.,-1.,0.));
#17752=DIRECTION('ref_axis',(0.309016994374948,0.,-0.951056516295154));
#17753=DIRECTION('center_axis',(0.,1.,0.));
#17754=DIRECTION('ref_axis',(1.,0.,0.));
#17755=DIRECTION('center_axis',(0.,-1.,0.));
#17756=DIRECTION('ref_axis',(0.156434465040231,0.,-0.987688340595138));
#17757=DIRECTION('center_axis',(0.,1.,0.));
#17758=DIRECTION('ref_axis',(1.,0.,0.));
#17759=DIRECTION('center_axis',(0.,-1.,0.));
#17760=DIRECTION('ref_axis',(6.12323399573677E-17,0.,-1.));
#17761=DIRECTION('center_axis',(0.,1.,0.));
#17762=DIRECTION('ref_axis',(1.,0.,0.));
#17763=DIRECTION('center_axis',(0.,-1.,0.));
#17764=DIRECTION('ref_axis',(-0.156434465040231,0.,-0.987688340595138));
#17765=DIRECTION('center_axis',(0.,1.,0.));
#17766=DIRECTION('ref_axis',(1.,0.,0.));
#17767=DIRECTION('center_axis',(0.,-1.,0.));
#17768=DIRECTION('ref_axis',(-0.309016994374947,0.,-0.951056516295154));
#17769=DIRECTION('center_axis',(0.,1.,0.));
#17770=DIRECTION('ref_axis',(1.,0.,0.));
#17771=DIRECTION('center_axis',(0.,-1.,0.));
#17772=DIRECTION('ref_axis',(-0.453990499739547,0.,-0.891006524188368));
#17773=DIRECTION('center_axis',(0.,1.,0.));
#17774=DIRECTION('ref_axis',(1.,0.,0.));
#17775=DIRECTION('center_axis',(0.,-1.,0.));
#17776=DIRECTION('ref_axis',(-0.587785252292473,0.,-0.809016994374947));
#17777=DIRECTION('center_axis',(0.,1.,0.));
#17778=DIRECTION('ref_axis',(1.,0.,0.));
#17779=DIRECTION('center_axis',(0.,-1.,0.));
#17780=DIRECTION('ref_axis',(-0.707106781186547,0.,-0.707106781186548));
#17781=DIRECTION('center_axis',(0.,1.,0.));
#17782=DIRECTION('ref_axis',(1.,0.,0.));
#17783=DIRECTION('center_axis',(0.,-1.,0.));
#17784=DIRECTION('ref_axis',(-0.809016994374947,0.,-0.587785252292473));
#17785=DIRECTION('center_axis',(0.,1.,0.));
#17786=DIRECTION('ref_axis',(1.,0.,0.));
#17787=DIRECTION('center_axis',(0.,-1.,0.));
#17788=DIRECTION('ref_axis',(-0.891006524188368,0.,-0.453990499739547));
#17789=DIRECTION('center_axis',(0.,1.,0.));
#17790=DIRECTION('ref_axis',(1.,0.,0.));
#17791=DIRECTION('center_axis',(0.,-1.,0.));
#17792=DIRECTION('ref_axis',(-0.951056516295154,0.,-0.309016994374948));
#17793=DIRECTION('center_axis',(0.,1.,0.));
#17794=DIRECTION('ref_axis',(1.,0.,0.));
#17795=DIRECTION('center_axis',(0.,-1.,0.));
#17796=DIRECTION('ref_axis',(-0.987688340595138,0.,-0.156434465040231));
#17797=DIRECTION('center_axis',(0.,1.,0.));
#17798=DIRECTION('ref_axis',(1.,0.,0.));
#17799=DIRECTION('center_axis',(0.,-1.,0.));
#17800=DIRECTION('ref_axis',(-1.,0.,-1.22464679914735E-16));
#17801=DIRECTION('center_axis',(0.,1.,0.));
#17802=DIRECTION('ref_axis',(1.,0.,0.));
#17803=DIRECTION('center_axis',(0.,-1.,0.));
#17804=DIRECTION('ref_axis',(-0.987688340595138,0.,0.156434465040231));
#17805=DIRECTION('center_axis',(0.,1.,0.));
#17806=DIRECTION('ref_axis',(1.,0.,0.));
#17807=DIRECTION('center_axis',(0.,-1.,0.));
#17808=DIRECTION('ref_axis',(-0.951056516295154,0.,0.309016994374947));
#17809=DIRECTION('center_axis',(0.,1.,0.));
#17810=DIRECTION('ref_axis',(1.,0.,0.));
#17811=DIRECTION('center_axis',(0.,-1.,0.));
#17812=DIRECTION('ref_axis',(-0.891006524188368,0.,0.453990499739547));
#17813=DIRECTION('center_axis',(0.,1.,0.));
#17814=DIRECTION('ref_axis',(1.,0.,0.));
#17815=DIRECTION('center_axis',(0.,-1.,0.));
#17816=DIRECTION('ref_axis',(-0.809016994374947,0.,0.587785252292473));
#17817=DIRECTION('center_axis',(0.,1.,0.));
#17818=DIRECTION('ref_axis',(1.,0.,0.));
#17819=DIRECTION('center_axis',(0.,-1.,0.));
#17820=DIRECTION('ref_axis',(-0.707106781186548,0.,0.707106781186547));
#17821=DIRECTION('center_axis',(0.,1.,0.));
#17822=DIRECTION('ref_axis',(1.,0.,0.));
#17823=DIRECTION('center_axis',(0.,-1.,0.));
#17824=DIRECTION('ref_axis',(-0.587785252292473,0.,0.809016994374947));
#17825=DIRECTION('center_axis',(0.,1.,0.));
#17826=DIRECTION('ref_axis',(1.,0.,0.));
#17827=DIRECTION('center_axis',(0.,-1.,0.));
#17828=DIRECTION('ref_axis',(-0.453990499739547,0.,0.891006524188368));
#17829=DIRECTION('center_axis',(0.,1.,0.));
#17830=DIRECTION('ref_axis',(1.,0.,0.));
#17831=DIRECTION('center_axis',(0.,-1.,0.));
#17832=DIRECTION('ref_axis',(-0.309016994374948,0.,0.951056516295154));
#17833=DIRECTION('center_axis',(0.,1.,0.));
#17834=DIRECTION('ref_axis',(1.,0.,0.));
#17835=DIRECTION('center_axis',(0.,-1.,0.));
#17836=DIRECTION('ref_axis',(-0.156434465040231,0.,0.987688340595138));
#17837=DIRECTION('center_axis',(0.,1.,0.));
#17838=DIRECTION('ref_axis',(1.,0.,0.));
#17839=DIRECTION('center_axis',(0.,-1.,0.));
#17840=DIRECTION('ref_axis',(-1.83697019872103E-16,0.,1.));
#17841=DIRECTION('center_axis',(0.,1.,0.));
#17842=DIRECTION('ref_axis',(1.,0.,0.));
#17843=DIRECTION('center_axis',(0.,-1.,0.));
#17844=DIRECTION('ref_axis',(0.156434465040231,0.,0.987688340595138));
#17845=DIRECTION('center_axis',(0.,1.,0.));
#17846=DIRECTION('ref_axis',(1.,0.,0.));
#17847=DIRECTION('center_axis',(0.,-1.,0.));
#17848=DIRECTION('ref_axis',(0.309016994374947,0.,0.951056516295154));
#17849=DIRECTION('center_axis',(0.,1.,0.));
#17850=DIRECTION('ref_axis',(1.,0.,0.));
#17851=DIRECTION('center_axis',(0.,-1.,0.));
#17852=DIRECTION('ref_axis',(0.453990499739547,0.,0.891006524188368));
#17853=DIRECTION('center_axis',(0.,1.,0.));
#17854=DIRECTION('ref_axis',(1.,0.,0.));
#17855=DIRECTION('center_axis',(0.,-1.,0.));
#17856=DIRECTION('ref_axis',(0.587785252292473,0.,0.809016994374948));
#17857=DIRECTION('center_axis',(0.,1.,0.));
#17858=DIRECTION('ref_axis',(1.,0.,0.));
#17859=DIRECTION('center_axis',(0.,-1.,0.));
#17860=DIRECTION('ref_axis',(0.707106781186547,0.,0.707106781186548));
#17861=DIRECTION('center_axis',(0.,1.,0.));
#17862=DIRECTION('ref_axis',(1.,0.,0.));
#17863=DIRECTION('center_axis',(0.,-1.,0.));
#17864=DIRECTION('ref_axis',(0.809016994374947,0.,0.587785252292473));
#17865=DIRECTION('center_axis',(0.,1.,0.));
#17866=DIRECTION('ref_axis',(1.,0.,0.));
#17867=DIRECTION('center_axis',(0.,-1.,0.));
#17868=DIRECTION('ref_axis',(0.891006524188368,0.,0.453990499739547));
#17869=DIRECTION('center_axis',(0.,1.,0.));
#17870=DIRECTION('ref_axis',(1.,0.,0.));
#17871=DIRECTION('center_axis',(0.,-1.,0.));
#17872=DIRECTION('ref_axis',(0.951056516295154,0.,0.309016994374948));
#17873=DIRECTION('center_axis',(0.,1.,0.));
#17874=DIRECTION('ref_axis',(1.,0.,0.));
#17875=DIRECTION('center_axis',(0.,1.,0.));
#17876=DIRECTION('ref_axis',(1.,0.,0.));
#17877=DIRECTION('center_axis',(0.,1.,0.));
#17878=DIRECTION('ref_axis',(1.,0.,0.));
#17879=DIRECTION('',(0.,-1.,0.));
#17880=DIRECTION('center_axis',(0.,1.,0.));
#17881=DIRECTION('ref_axis',(1.,0.,0.));
#17882=DIRECTION('center_axis',(0.,1.,0.));
#17883=DIRECTION('ref_axis',(-0.987688340595137,0.,-0.156434465040233));
#17884=DIRECTION('',(0.,-1.,0.));
#17885=DIRECTION('',(0.,1.,0.));
#17886=DIRECTION('center_axis',(0.,1.,0.));
#17887=DIRECTION('ref_axis',(1.,0.,0.));
#17888=DIRECTION('',(0.,-1.,0.));
#17889=DIRECTION('center_axis',(0.,1.,0.));
#17890=DIRECTION('ref_axis',(-0.951056516295153,0.,-0.309016994374949));
#17891=DIRECTION('',(0.,1.,0.));
#17892=DIRECTION('center_axis',(0.,1.,0.));
#17893=DIRECTION('ref_axis',(1.,0.,0.));
#17894=DIRECTION('',(0.,-1.,0.));
#17895=DIRECTION('center_axis',(0.,1.,0.));
#17896=DIRECTION('ref_axis',(-0.891006524188368,0.,-0.453990499739547));
#17897=DIRECTION('',(0.,1.,0.));
#17898=DIRECTION('center_axis',(0.,1.,0.));
#17899=DIRECTION('ref_axis',(1.,0.,0.));
#17900=DIRECTION('',(0.,-1.,0.));
#17901=DIRECTION('center_axis',(0.,1.,0.));
#17902=DIRECTION('ref_axis',(-0.809016994374948,0.,-0.587785252292473));
#17903=DIRECTION('',(0.,1.,0.));
#17904=DIRECTION('center_axis',(0.,1.,0.));
#17905=DIRECTION('ref_axis',(1.,0.,0.));
#17906=DIRECTION('',(0.,-1.,0.));
#17907=DIRECTION('center_axis',(0.,1.,0.));
#17908=DIRECTION('ref_axis',(-0.707106781186547,0.,-0.707106781186548));
#17909=DIRECTION('',(0.,1.,0.));
#17910=DIRECTION('center_axis',(0.,1.,0.));
#17911=DIRECTION('ref_axis',(1.,0.,0.));
#17912=DIRECTION('',(0.,-1.,0.));
#17913=DIRECTION('center_axis',(0.,1.,0.));
#17914=DIRECTION('ref_axis',(-0.587785252292474,0.,-0.809016994374947));
#17915=DIRECTION('',(0.,1.,0.));
#17916=DIRECTION('center_axis',(0.,1.,0.));
#17917=DIRECTION('ref_axis',(1.,0.,0.));
#17918=DIRECTION('',(0.,-1.,0.));
#17919=DIRECTION('center_axis',(0.,1.,0.));
#17920=DIRECTION('ref_axis',(-0.453990499739547,0.,-0.891006524188368));
#17921=DIRECTION('',(0.,1.,0.));
#17922=DIRECTION('center_axis',(0.,1.,0.));
#17923=DIRECTION('ref_axis',(1.,0.,0.));
#17924=DIRECTION('',(0.,-1.,0.));
#17925=DIRECTION('center_axis',(0.,1.,0.));
#17926=DIRECTION('ref_axis',(-0.309016994374948,0.,-0.951056516295153));
#17927=DIRECTION('',(0.,1.,0.));
#17928=DIRECTION('center_axis',(0.,1.,0.));
#17929=DIRECTION('ref_axis',(1.,0.,0.));
#17930=DIRECTION('',(0.,-1.,0.));
#17931=DIRECTION('center_axis',(0.,1.,0.));
#17932=DIRECTION('ref_axis',(-0.156434465040232,0.,-0.987688340595138));
#17933=DIRECTION('',(0.,1.,0.));
#17934=DIRECTION('center_axis',(0.,1.,0.));
#17935=DIRECTION('ref_axis',(1.,0.,0.));
#17936=DIRECTION('',(0.,-1.,0.));
#17937=DIRECTION('center_axis',(0.,1.,0.));
#17938=DIRECTION('ref_axis',(3.06161699786838E-16,0.,-1.));
#17939=DIRECTION('',(0.,1.,0.));
#17940=DIRECTION('center_axis',(0.,1.,0.));
#17941=DIRECTION('ref_axis',(1.,0.,0.));
#17942=DIRECTION('',(0.,-1.,0.));
#17943=DIRECTION('center_axis',(0.,1.,0.));
#17944=DIRECTION('ref_axis',(0.156434465040233,0.,-0.987688340595138));
#17945=DIRECTION('',(0.,1.,0.));
#17946=DIRECTION('center_axis',(0.,1.,0.));
#17947=DIRECTION('ref_axis',(1.,0.,0.));
#17948=DIRECTION('',(0.,-1.,0.));
#17949=DIRECTION('center_axis',(0.,1.,0.));
#17950=DIRECTION('ref_axis',(0.309016994374946,0.,-0.951056516295154));
#17951=DIRECTION('',(0.,1.,0.));
#17952=DIRECTION('center_axis',(0.,1.,0.));
#17953=DIRECTION('ref_axis',(1.,0.,0.));
#17954=DIRECTION('',(0.,-1.,0.));
#17955=DIRECTION('center_axis',(0.,1.,0.));
#17956=DIRECTION('ref_axis',(0.453990499739547,0.,-0.891006524188368));
#17957=DIRECTION('',(0.,1.,0.));
#17958=DIRECTION('center_axis',(0.,1.,0.));
#17959=DIRECTION('ref_axis',(1.,0.,0.));
#17960=DIRECTION('',(0.,-1.,0.));
#17961=DIRECTION('center_axis',(0.,1.,0.));
#17962=DIRECTION('ref_axis',(0.587785252292473,0.,-0.809016994374947));
#17963=DIRECTION('',(0.,1.,0.));
#17964=DIRECTION('center_axis',(0.,1.,0.));
#17965=DIRECTION('ref_axis',(1.,0.,0.));
#17966=DIRECTION('',(0.,-1.,0.));
#17967=DIRECTION('center_axis',(0.,1.,0.));
#17968=DIRECTION('ref_axis',(0.707106781186548,0.,-0.707106781186547));
#17969=DIRECTION('',(0.,1.,0.));
#17970=DIRECTION('center_axis',(0.,1.,0.));
#17971=DIRECTION('ref_axis',(1.,0.,0.));
#17972=DIRECTION('',(0.,-1.,0.));
#17973=DIRECTION('center_axis',(0.,1.,0.));
#17974=DIRECTION('ref_axis',(0.809016994374946,0.,-0.587785252292475));
#17975=DIRECTION('',(0.,1.,0.));
#17976=DIRECTION('center_axis',(0.,1.,0.));
#17977=DIRECTION('ref_axis',(1.,0.,0.));
#17978=DIRECTION('',(0.,-1.,0.));
#17979=DIRECTION('center_axis',(0.,1.,0.));
#17980=DIRECTION('ref_axis',(0.891006524188368,0.,-0.453990499739547));
#17981=DIRECTION('',(0.,1.,0.));
#17982=DIRECTION('center_axis',(0.,1.,0.));
#17983=DIRECTION('ref_axis',(1.,0.,0.));
#17984=DIRECTION('',(0.,-1.,0.));
#17985=DIRECTION('center_axis',(0.,1.,0.));
#17986=DIRECTION('ref_axis',(0.951056516295154,0.,-0.309016994374946));
#17987=DIRECTION('',(0.,1.,0.));
#17988=DIRECTION('center_axis',(0.,1.,0.));
#17989=DIRECTION('ref_axis',(1.,0.,0.));
#17990=DIRECTION('',(0.,-1.,0.));
#17991=DIRECTION('center_axis',(0.,1.,0.));
#17992=DIRECTION('ref_axis',(0.987688340595138,0.,-0.156434465040232));
#17993=DIRECTION('',(0.,1.,0.));
#17994=DIRECTION('center_axis',(0.,1.,0.));
#17995=DIRECTION('ref_axis',(1.,0.,0.));
#17996=DIRECTION('',(0.,-1.,0.));
#17997=DIRECTION('center_axis',(0.,1.,0.));
#17998=DIRECTION('ref_axis',(1.,0.,2.44929359829471E-16));
#17999=DIRECTION('',(0.,1.,0.));
#18000=DIRECTION('center_axis',(0.,1.,0.));
#18001=DIRECTION('ref_axis',(1.,0.,0.));
#18002=DIRECTION('',(0.,-1.,0.));
#18003=DIRECTION('center_axis',(0.,1.,0.));
#18004=DIRECTION('ref_axis',(0.987688340595137,0.,0.156434465040232));
#18005=DIRECTION('',(0.,1.,0.));
#18006=DIRECTION('center_axis',(0.,1.,0.));
#18007=DIRECTION('ref_axis',(1.,0.,0.));
#18008=DIRECTION('',(0.,-1.,0.));
#18009=DIRECTION('center_axis',(0.,1.,0.));
#18010=DIRECTION('ref_axis',(0.951056516295154,0.,0.309016994374946));
#18011=DIRECTION('',(0.,1.,0.));
#18012=DIRECTION('center_axis',(0.,1.,0.));
#18013=DIRECTION('ref_axis',(1.,0.,0.));
#18014=DIRECTION('',(0.,-1.,0.));
#18015=DIRECTION('center_axis',(0.,1.,0.));
#18016=DIRECTION('ref_axis',(0.891006524188368,0.,0.453990499739547));
#18017=DIRECTION('',(0.,1.,0.));
#18018=DIRECTION('center_axis',(0.,1.,0.));
#18019=DIRECTION('ref_axis',(1.,0.,0.));
#18020=DIRECTION('',(0.,-1.,0.));
#18021=DIRECTION('center_axis',(0.,1.,0.));
#18022=DIRECTION('ref_axis',(0.809016994374947,0.,0.587785252292473));
#18023=DIRECTION('',(0.,1.,0.));
#18024=DIRECTION('center_axis',(0.,1.,0.));
#18025=DIRECTION('ref_axis',(1.,0.,0.));
#18026=DIRECTION('',(0.,-1.,0.));
#18027=DIRECTION('center_axis',(0.,1.,0.));
#18028=DIRECTION('ref_axis',(0.707106781186547,0.,0.707106781186548));
#18029=DIRECTION('',(0.,1.,0.));
#18030=DIRECTION('center_axis',(0.,1.,0.));
#18031=DIRECTION('ref_axis',(1.,0.,0.));
#18032=DIRECTION('',(0.,-1.,0.));
#18033=DIRECTION('center_axis',(0.,1.,0.));
#18034=DIRECTION('ref_axis',(0.587785252292475,0.,0.809016994374946));
#18035=DIRECTION('',(0.,1.,0.));
#18036=DIRECTION('center_axis',(0.,1.,0.));
#18037=DIRECTION('ref_axis',(1.,0.,0.));
#18038=DIRECTION('',(0.,-1.,0.));
#18039=DIRECTION('center_axis',(0.,1.,0.));
#18040=DIRECTION('ref_axis',(0.453990499739547,0.,0.891006524188368));
#18041=DIRECTION('',(0.,1.,0.));
#18042=DIRECTION('center_axis',(0.,1.,0.));
#18043=DIRECTION('ref_axis',(1.,0.,0.));
#18044=DIRECTION('',(0.,-1.,0.));
#18045=DIRECTION('center_axis',(0.,1.,0.));
#18046=DIRECTION('ref_axis',(0.309016994374946,0.,0.951056516295154));
#18047=DIRECTION('',(0.,1.,0.));
#18048=DIRECTION('center_axis',(0.,1.,0.));
#18049=DIRECTION('ref_axis',(1.,0.,0.));
#18050=DIRECTION('',(0.,-1.,0.));
#18051=DIRECTION('center_axis',(0.,1.,0.));
#18052=DIRECTION('ref_axis',(0.156434465040232,0.,0.987688340595138));
#18053=DIRECTION('',(0.,1.,0.));
#18054=DIRECTION('center_axis',(0.,1.,0.));
#18055=DIRECTION('ref_axis',(1.,0.,0.));
#18056=DIRECTION('',(0.,-1.,0.));
#18057=DIRECTION('center_axis',(0.,1.,0.));
#18058=DIRECTION('ref_axis',(-1.83697019872103E-16,0.,1.));
#18059=DIRECTION('',(0.,1.,0.));
#18060=DIRECTION('center_axis',(0.,1.,0.));
#18061=DIRECTION('ref_axis',(1.,0.,0.));
#18062=DIRECTION('',(0.,-1.,0.));
#18063=DIRECTION('center_axis',(0.,1.,0.));
#18064=DIRECTION('ref_axis',(-0.156434465040232,0.,0.987688340595138));
#18065=DIRECTION('',(0.,1.,0.));
#18066=DIRECTION('center_axis',(0.,1.,0.));
#18067=DIRECTION('ref_axis',(1.,0.,0.));
#18068=DIRECTION('',(0.,-1.,0.));
#18069=DIRECTION('center_axis',(0.,1.,0.));
#18070=DIRECTION('ref_axis',(-0.309016994374946,0.,0.951056516295154));
#18071=DIRECTION('',(0.,1.,0.));
#18072=DIRECTION('center_axis',(0.,1.,0.));
#18073=DIRECTION('ref_axis',(1.,0.,0.));
#18074=DIRECTION('',(0.,-1.,0.));
#18075=DIRECTION('center_axis',(0.,1.,0.));
#18076=DIRECTION('ref_axis',(-0.453990499739549,0.,0.891006524188367));
#18077=DIRECTION('',(0.,1.,0.));
#18078=DIRECTION('center_axis',(0.,1.,0.));
#18079=DIRECTION('ref_axis',(1.,0.,0.));
#18080=DIRECTION('',(0.,-1.,0.));
#18081=DIRECTION('center_axis',(0.,1.,0.));
#18082=DIRECTION('ref_axis',(-0.587785252292474,0.,0.809016994374947));
#18083=DIRECTION('',(0.,1.,0.));
#18084=DIRECTION('center_axis',(0.,1.,0.));
#18085=DIRECTION('ref_axis',(1.,0.,0.));
#18086=DIRECTION('',(0.,-1.,0.));
#18087=DIRECTION('center_axis',(0.,1.,0.));
#18088=DIRECTION('ref_axis',(-0.707106781186548,0.,0.707106781186547));
#18089=DIRECTION('',(0.,1.,0.));
#18090=DIRECTION('center_axis',(0.,1.,0.));
#18091=DIRECTION('ref_axis',(1.,0.,0.));
#18092=DIRECTION('',(0.,-1.,0.));
#18093=DIRECTION('center_axis',(0.,1.,0.));
#18094=DIRECTION('ref_axis',(-0.809016994374947,0.,0.587785252292474));
#18095=DIRECTION('',(0.,1.,0.));
#18096=DIRECTION('center_axis',(0.,1.,0.));
#18097=DIRECTION('ref_axis',(1.,0.,0.));
#18098=DIRECTION('',(0.,-1.,0.));
#18099=DIRECTION('center_axis',(0.,1.,0.));
#18100=DIRECTION('ref_axis',(-0.891006524188368,0.,0.453990499739547));
#18101=DIRECTION('',(0.,1.,0.));
#18102=DIRECTION('center_axis',(0.,1.,0.));
#18103=DIRECTION('ref_axis',(1.,0.,0.));
#18104=DIRECTION('',(0.,-1.,0.));
#18105=DIRECTION('center_axis',(0.,1.,0.));
#18106=DIRECTION('ref_axis',(-0.951056516295154,0.,0.309016994374948));
#18107=DIRECTION('',(0.,1.,0.));
#18108=DIRECTION('center_axis',(0.,1.,0.));
#18109=DIRECTION('ref_axis',(1.,0.,0.));
#18110=DIRECTION('',(0.,-1.,0.));
#18111=DIRECTION('center_axis',(0.,1.,0.));
#18112=DIRECTION('ref_axis',(-0.987688340595137,0.,0.156434465040233));
#18113=DIRECTION('',(0.,1.,0.));
#18114=DIRECTION('center_axis',(0.,1.,0.));
#18115=DIRECTION('ref_axis',(1.,0.,0.));
#18116=DIRECTION('',(0.,1.,0.));
#18117=DIRECTION('center_axis',(0.,1.,0.));
#18118=DIRECTION('ref_axis',(-1.,0.,-1.22464679914735E-16));
#18119=DIRECTION('',(0.,-1.,0.));
#18120=DIRECTION('center_axis',(0.,1.,0.));
#18121=DIRECTION('ref_axis',(1.,0.,0.));
#22245=CARTESIAN_POINT('',(0.,0.,0.));
#22246=CARTESIAN_POINT('Origin',(0.,-0.5,0.));
#22247=CARTESIAN_POINT('',(-1.,-0.375,-6.12323399573677E-17));
#22248=CARTESIAN_POINT('',(-0.992156741649222,-0.5,0.125));
#22249=CARTESIAN_POINT('Ctrl Pts',(-1.,-0.375,-1.00613961606655E-16));
#22250=CARTESIAN_POINT('Ctrl Pts',(-1.,-0.375,0.0157128711428661));
#22251=CARTESIAN_POINT('Ctrl Pts',(-0.999591823858855,-0.378143583103513,
0.0324619190698278));
#22252=CARTESIAN_POINT('Ctrl Pts',(-0.998116453123232,-0.390905426591754,
0.0632545375991437));
#22253=CARTESIAN_POINT('Ctrl Pts',(-0.997070068816062,-0.400522781657727,
0.0772994769543643));
#22254=CARTESIAN_POINT('Ctrl Pts',(-0.995102104277285,-0.422700615683787,
0.0994773109804239));
#22255=CARTESIAN_POINT('Ctrl Pts',(-0.994052129228928,-0.436745514765346,
0.109094593469654));
#22256=CARTESIAN_POINT('Ctrl Pts',(-0.99256853061881,-0.467537996927464,
0.121856383722779));
#22257=CARTESIAN_POINT('Ctrl Pts',(-0.992156741649222,-0.484286997589363,
0.125));
#22258=CARTESIAN_POINT('Ctrl Pts',(-0.992156741649222,-0.5,0.125));
#22259=CARTESIAN_POINT('',(-1.,-0.625,-6.12323399573677E-17));
#22260=CARTESIAN_POINT('Ctrl Pts',(-1.,-0.625,-4.5102810375397E-17));
#22261=CARTESIAN_POINT('Ctrl Pts',(-1.,-0.625,-0.0157128711428662));
#22262=CARTESIAN_POINT('Ctrl Pts',(-0.999591823858855,-0.621856416896487,
-0.032461919069828));
#22263=CARTESIAN_POINT('Ctrl Pts',(-0.998116453123232,-0.609094573408246,
-0.0632545375991439));
#22264=CARTESIAN_POINT('Ctrl Pts',(-0.997070068816062,-0.599477218342273,
-0.0772994769543645));
#22265=CARTESIAN_POINT('Ctrl Pts',(-0.995102104277285,-0.577299384316213,
-0.0994773109804241));
#22266=CARTESIAN_POINT('Ctrl Pts',(-0.994052129228928,-0.563254485234654,
-0.109094593469655));
#22267=CARTESIAN_POINT('Ctrl Pts',(-0.99256853061881,-0.532462003072536,
-0.121856383722779));
#22268=CARTESIAN_POINT('Ctrl Pts',(-0.992156741649221,-0.515713002410637,
-0.125));
#22269=CARTESIAN_POINT('Ctrl Pts',(-0.992156741649221,-0.484286997589363,
-0.125));
#22270=CARTESIAN_POINT('Ctrl Pts',(-0.99256853061881,-0.467537996927464,
-0.121856383722779));
#22271=CARTESIAN_POINT('Ctrl Pts',(-0.994052129228928,-0.436745514765346,
-0.109094593469655));
#22272=CARTESIAN_POINT('Ctrl Pts',(-0.995102104277285,-0.422700615683787,
-0.0994773109804241));
#22273=CARTESIAN_POINT('Ctrl Pts',(-0.997070068816062,-0.400522781657728,
-0.0772994769543645));
#22274=CARTESIAN_POINT('Ctrl Pts',(-0.998116453123232,-0.390905426591754,
-0.063254537599144));
#22275=CARTESIAN_POINT('Ctrl Pts',(-0.999591823858855,-0.378143583103513,
-0.0324619190698281));
#22276=CARTESIAN_POINT('Ctrl Pts',(-1.,-0.375,-0.0157128711428663));
#22277=CARTESIAN_POINT('Ctrl Pts',(-1.,-0.375,-9.36750677027476E-17));
#22278=CARTESIAN_POINT('Ctrl Pts',(-0.992156741649222,-0.5,0.125));
#22279=CARTESIAN_POINT('Ctrl Pts',(-0.992156741649222,-0.515713002410637,
0.125));
#22280=CARTESIAN_POINT('Ctrl Pts',(-0.99256853061881,-0.532462003072536,
0.121856383722779));
#22281=CARTESIAN_POINT('Ctrl Pts',(-0.994052129228928,-0.563254485234654,
0.109094593469654));
#22282=CARTESIAN_POINT('Ctrl Pts',(-0.995102104277285,-0.577299384316213,
0.0994773109804241));
#22283=CARTESIAN_POINT('Ctrl Pts',(-0.997070068816062,-0.599477218342273,
0.0772994769543644));
#22284=CARTESIAN_POINT('Ctrl Pts',(-0.998116453123232,-0.609094573408246,
0.0632545375991438));
#22285=CARTESIAN_POINT('Ctrl Pts',(-0.999591823858855,-0.621856416896487,
0.0324619190698279));
#22286=CARTESIAN_POINT('Ctrl Pts',(-1.,-0.625,0.0157128711428661));
#22287=CARTESIAN_POINT('Ctrl Pts',(-1.,-0.625,-4.85722573273506E-17));
#22288=CARTESIAN_POINT('',(-0.586834729715275,-0.5,0.125));
#22289=CARTESIAN_POINT('',(-7.65404249467096E-18,-0.5,0.125));
#22290=CARTESIAN_POINT('',(-0.6,-0.625,1.24532753107453E-17));
#22291=CARTESIAN_POINT('Ctrl Pts',(-0.6,-0.625,-4.16333634234434E-17));
#22292=CARTESIAN_POINT('Ctrl Pts',(-0.6,-0.625,0.0157444828659572));
#22293=CARTESIAN_POINT('Ctrl Pts',(-0.599317707212167,-0.621844041497889,
0.0325072544867633));
#22294=CARTESIAN_POINT('Ctrl Pts',(-0.596852269967858,-0.609072857638709,
0.0632914182239686));
#22295=CARTESIAN_POINT('Ctrl Pts',(-0.59510289473619,-0.599460146728784,
0.077316548567853));
#22296=CARTESIAN_POINT('Ctrl Pts',(-0.591804743154611,-0.577315815675743,
0.0994608796208941));
#22297=CARTESIAN_POINT('Ctrl Pts',(-0.590038488226116,-0.563290995658393,
0.109073016834181));
#22298=CARTESIAN_POINT('Ctrl Pts',(-0.587534197873268,-0.532507913768158,
0.121843784097853));
#22299=CARTESIAN_POINT('Ctrl Pts',(-0.586834729715275,-0.515745525063995,
0.125));
#22300=CARTESIAN_POINT('Ctrl Pts',(-0.586834729715275,-0.5,0.125));
#22301=CARTESIAN_POINT('',(-0.586834729715275,-0.5,-0.125));
#22302=CARTESIAN_POINT('Ctrl Pts',(-0.586834729715275,-0.5,-0.125));
#22303=CARTESIAN_POINT('Ctrl Pts',(-0.586834729715275,-0.515745525063995,
-0.125));
#22304=CARTESIAN_POINT('Ctrl Pts',(-0.587534197873268,-0.532507913768158,
-0.121843784097853));
#22305=CARTESIAN_POINT('Ctrl Pts',(-0.590038488226116,-0.563290995658393,
-0.109073016834181));
#22306=CARTESIAN_POINT('Ctrl Pts',(-0.591804743154611,-0.577315815675743,
-0.0994608796208942));
#22307=CARTESIAN_POINT('Ctrl Pts',(-0.59510289473619,-0.599460146728784,
-0.0773165485678531));
#22308=CARTESIAN_POINT('Ctrl Pts',(-0.596852269967858,-0.609072857638709,
-0.0632914182239687));
#22309=CARTESIAN_POINT('Ctrl Pts',(-0.599317707212167,-0.621844041497889,
-0.0325072544867635));
#22310=CARTESIAN_POINT('Ctrl Pts',(-0.6,-0.625,-0.0157444828659573));
#22311=CARTESIAN_POINT('Ctrl Pts',(-0.6,-0.625,-5.20417042793042E-17));
#22312=CARTESIAN_POINT('',(-0.6,-0.375,3.50046804984438E-17));
#22313=CARTESIAN_POINT('Ctrl Pts',(-0.6,-0.375,-3.46944695195361E-18));
#22314=CARTESIAN_POINT('Ctrl Pts',(-0.6,-0.375,-0.0157444828659572));
#22315=CARTESIAN_POINT('Ctrl Pts',(-0.599317707212167,-0.378155958502111,
-0.0325072544867634));
#22316=CARTESIAN_POINT('Ctrl Pts',(-0.596852269967858,-0.390927142361291,
-0.0632914182239686));
#22317=CARTESIAN_POINT('Ctrl Pts',(-0.59510289473619,-0.400539853271216,
-0.077316548567853));
#22318=CARTESIAN_POINT('Ctrl Pts',(-0.591804743154611,-0.422684184324257,
-0.0994608796208942));
#22319=CARTESIAN_POINT('Ctrl Pts',(-0.590038488226116,-0.436709004341607,
-0.109073016834181));
#22320=CARTESIAN_POINT('Ctrl Pts',(-0.587534197873268,-0.467492086231842,
-0.121843784097853));
#22321=CARTESIAN_POINT('Ctrl Pts',(-0.586834729715275,-0.484254474936005,
-0.125));
#22322=CARTESIAN_POINT('Ctrl Pts',(-0.586834729715275,-0.5,-0.125));
#22323=CARTESIAN_POINT('Ctrl Pts',(-0.586834729715275,-0.5,0.125));
#22324=CARTESIAN_POINT('Ctrl Pts',(-0.586834729715275,-0.484254474936005,
0.125));
#22325=CARTESIAN_POINT('Ctrl Pts',(-0.587534197873268,-0.467492086231842,
0.121843784097853));
#22326=CARTESIAN_POINT('Ctrl Pts',(-0.590038488226116,-0.436709004341607,
0.109073016834181));
#22327=CARTESIAN_POINT('Ctrl Pts',(-0.591804743154611,-0.422684184324257,
0.0994608796208941));
#22328=CARTESIAN_POINT('Ctrl Pts',(-0.59510289473619,-0.400539853271216,
0.077316548567853));
#22329=CARTESIAN_POINT('Ctrl Pts',(-0.596852269967858,-0.390927142361291,
0.0632914182239686));
#22330=CARTESIAN_POINT('Ctrl Pts',(-0.599317707212167,-0.378155958502111,
0.0325072544867634));
#22331=CARTESIAN_POINT('Ctrl Pts',(-0.6,-0.375,0.0157444828659572));
#22332=CARTESIAN_POINT('Ctrl Pts',(-0.6,-0.375,-2.42861286636753E-17));
#22333=CARTESIAN_POINT('Origin',(0.,-0.5,0.));
#22334=CARTESIAN_POINT('',(0.586834729715275,-0.5,-0.125));
#22335=CARTESIAN_POINT('',(0.586834729715275,-0.5,0.125));
#22336=CARTESIAN_POINT('Ctrl Pts',(0.586834729715275,-0.5,-0.125));
#22337=CARTESIAN_POINT('Ctrl Pts',(0.586834729715275,-0.484254474936005,
-0.125));
#22338=CARTESIAN_POINT('Ctrl Pts',(0.587534197873268,-0.467492086231842,
-0.121843784097853));
#22339=CARTESIAN_POINT('Ctrl Pts',(0.590038488226116,-0.436709004341607,
-0.109073016834181));
#22340=CARTESIAN_POINT('Ctrl Pts',(0.591804743154611,-0.422684184324257,
-0.0994608796208941));
#22341=CARTESIAN_POINT('Ctrl Pts',(0.59510289473619,-0.400539853271216,
-0.0773165485678529));
#22342=CARTESIAN_POINT('Ctrl Pts',(0.596852269967858,-0.390927142361291,
-0.0632914182239686));
#22343=CARTESIAN_POINT('Ctrl Pts',(0.599317707212167,-0.378155958502111,
-0.0325072544867633));
#22344=CARTESIAN_POINT('Ctrl Pts',(0.6,-0.375,-0.0157444828659572));
#22345=CARTESIAN_POINT('Ctrl Pts',(0.6,-0.375,0.0157444828659573));
#22346=CARTESIAN_POINT('Ctrl Pts',(0.599317707212167,-0.378155958502111,
0.0325072544867635));
#22347=CARTESIAN_POINT('Ctrl Pts',(0.596852269967858,-0.390927142361291,
0.0632914182239687));
#22348=CARTESIAN_POINT('Ctrl Pts',(0.59510289473619,-0.400539853271216,
0.0773165485678531));
#22349=CARTESIAN_POINT('Ctrl Pts',(0.591804743154611,-0.422684184324257,
0.0994608796208942));
#22350=CARTESIAN_POINT('Ctrl Pts',(0.590038488226116,-0.436709004341607,
0.109073016834181));
#22351=CARTESIAN_POINT('Ctrl Pts',(0.587534197873268,-0.467492086231842,
0.121843784097853));
#22352=CARTESIAN_POINT('Ctrl Pts',(0.586834729715275,-0.484254474936005,
0.125));
#22353=CARTESIAN_POINT('Ctrl Pts',(0.586834729715275,-0.5,0.125));
#22354=CARTESIAN_POINT('Ctrl Pts',(0.586834729715275,-0.5,0.125));
#22355=CARTESIAN_POINT('Ctrl Pts',(0.586834729715275,-0.515745525063995,
0.125));
#22356=CARTESIAN_POINT('Ctrl Pts',(0.587534197873268,-0.532507913768158,
0.121843784097853));
#22357=CARTESIAN_POINT('Ctrl Pts',(0.590038488226116,-0.563290995658393,
0.109073016834181));
#22358=CARTESIAN_POINT('Ctrl Pts',(0.591804743154611,-0.577315815675743,
0.0994608796208942));
#22359=CARTESIAN_POINT('Ctrl Pts',(0.59510289473619,-0.599460146728784,
0.077316548567853));
#22360=CARTESIAN_POINT('Ctrl Pts',(0.596852269967858,-0.609072857638709,
0.0632914182239688));
#22361=CARTESIAN_POINT('Ctrl Pts',(0.599317707212167,-0.621844041497889,
0.0325072544867635));
#22362=CARTESIAN_POINT('Ctrl Pts',(0.6,-0.625,0.0157444828659573));
#22363=CARTESIAN_POINT('Ctrl Pts',(0.6,-0.625,-0.0157444828659572));
#22364=CARTESIAN_POINT('Ctrl Pts',(0.599317707212167,-0.621844041497889,
-0.0325072544867633));
#22365=CARTESIAN_POINT('Ctrl Pts',(0.596852269967858,-0.609072857638709,
-0.0632914182239685));
#22366=CARTESIAN_POINT('Ctrl Pts',(0.59510289473619,-0.599460146728784,
-0.077316548567853));
#22367=CARTESIAN_POINT('Ctrl Pts',(0.591804743154611,-0.577315815675743,
-0.0994608796208941));
#22368=CARTESIAN_POINT('Ctrl Pts',(0.590038488226116,-0.563290995658393,
-0.10907301683418));
#22369=CARTESIAN_POINT('Ctrl Pts',(0.587534197873268,-0.532507913768158,
-0.121843784097853));
#22370=CARTESIAN_POINT('Ctrl Pts',(0.586834729715275,-0.515745525063995,
-0.125));
#22371=CARTESIAN_POINT('Ctrl Pts',(0.586834729715275,-0.5,-0.125));
#22372=CARTESIAN_POINT('',(0.992156741649222,-0.5,0.125));
#22373=CARTESIAN_POINT('',(-7.65404249467096E-18,-0.5,0.125));
#22374=CARTESIAN_POINT('',(1.,-0.625,6.12323399573677E-17));
#22375=CARTESIAN_POINT('Ctrl Pts',(1.,-0.625,7.28583859910259E-17));
#22376=CARTESIAN_POINT('Ctrl Pts',(1.,-0.625,0.0157128711428663));
#22377=CARTESIAN_POINT('Ctrl Pts',(0.999591823858855,-0.621856416896487,
0.032461919069828));
#22378=CARTESIAN_POINT('Ctrl Pts',(0.998116453123232,-0.609094573408246,
0.0632545375991439));
#22379=CARTESIAN_POINT('Ctrl Pts',(0.997070068816062,-0.599477218342273,
0.0772994769543645));
#22380=CARTESIAN_POINT('Ctrl Pts',(0.995102104277285,-0.577299384316213,
0.0994773109804242));
#22381=CARTESIAN_POINT('Ctrl Pts',(0.994052129228928,-0.563254485234654,
0.109094593469655));
#22382=CARTESIAN_POINT('Ctrl Pts',(0.99256853061881,-0.532462003072536,
0.121856383722779));
#22383=CARTESIAN_POINT('Ctrl Pts',(0.992156741649222,-0.515713002410637,
0.125));
#22384=CARTESIAN_POINT('Ctrl Pts',(0.992156741649222,-0.5,0.125));
#22385=CARTESIAN_POINT('',(1.,-0.375,6.12323399573677E-17));
#22386=CARTESIAN_POINT('Ctrl Pts',(1.,-0.375,2.08166817117217E-17));
#22387=CARTESIAN_POINT('Ctrl Pts',(1.,-0.375,-0.0157128711428662));
#22388=CARTESIAN_POINT('Ctrl Pts',(0.999591823858855,-0.378143583103513,
-0.032461919069828));
#22389=CARTESIAN_POINT('Ctrl Pts',(0.998116453123232,-0.390905426591754,
-0.0632545375991438));
#22390=CARTESIAN_POINT('Ctrl Pts',(0.997070068816062,-0.400522781657728,
-0.0772994769543644));
#22391=CARTESIAN_POINT('Ctrl Pts',(0.995102104277285,-0.422700615683787,
-0.099477310980424));
#22392=CARTESIAN_POINT('Ctrl Pts',(0.994052129228928,-0.436745514765346,
-0.109094593469654));
#22393=CARTESIAN_POINT('Ctrl Pts',(0.99256853061881,-0.467537996927464,
-0.121856383722779));
#22394=CARTESIAN_POINT('Ctrl Pts',(0.992156741649222,-0.484286997589363,
-0.125));
#22395=CARTESIAN_POINT('Ctrl Pts',(0.992156741649222,-0.515713002410637,
-0.125));
#22396=CARTESIAN_POINT('Ctrl Pts',(0.99256853061881,-0.532462003072536,
-0.121856383722779));
#22397=CARTESIAN_POINT('Ctrl Pts',(0.994052129228928,-0.563254485234654,
-0.109094593469654));
#22398=CARTESIAN_POINT('Ctrl Pts',(0.995102104277285,-0.577299384316213,
-0.099477310980424));
#22399=CARTESIAN_POINT('Ctrl Pts',(0.997070068816062,-0.599477218342273,
-0.0772994769543643));
#22400=CARTESIAN_POINT('Ctrl Pts',(0.998116453123232,-0.609094573408246,
-0.0632545375991438));
#22401=CARTESIAN_POINT('Ctrl Pts',(0.999591823858855,-0.621856416896487,
-0.0324619190698279));
#22402=CARTESIAN_POINT('Ctrl Pts',(1.,-0.625,-0.0157128711428661));
#22403=CARTESIAN_POINT('Ctrl Pts',(1.,-0.625,8.32667268468867E-17));
#22404=CARTESIAN_POINT('Ctrl Pts',(0.992156741649222,-0.5,0.125));
#22405=CARTESIAN_POINT('Ctrl Pts',(0.992156741649222,-0.484286997589363,
0.125));
#22406=CARTESIAN_POINT('Ctrl Pts',(0.99256853061881,-0.467537996927464,
0.121856383722779));
#22407=CARTESIAN_POINT('Ctrl Pts',(0.994052129228928,-0.436745514765346,
0.109094593469654));
#22408=CARTESIAN_POINT('Ctrl Pts',(0.995102104277285,-0.422700615683787,
0.0994773109804241));
#22409=CARTESIAN_POINT('Ctrl Pts',(0.997070068816062,-0.400522781657727,
0.0772994769543644));
#22410=CARTESIAN_POINT('Ctrl Pts',(0.998116453123232,-0.390905426591754,
0.0632545375991438));
#22411=CARTESIAN_POINT('Ctrl Pts',(0.999591823858855,-0.378143583103513,
0.0324619190698279));
#22412=CARTESIAN_POINT('Ctrl Pts',(1.,-0.375,0.0157128711428662));
#22413=CARTESIAN_POINT('Ctrl Pts',(1.,-0.375,2.77555756156289E-17));
#22414=CARTESIAN_POINT('Origin',(0.,-0.1,0.));
#22415=CARTESIAN_POINT('',(-1.,-0.9,1.22464679914735E-16));
#22416=CARTESIAN_POINT('Origin',(0.,-0.9,0.));
#22417=CARTESIAN_POINT('',(-1.,-0.1,-1.22464679914735E-16));
#22418=CARTESIAN_POINT('',(-1.,-0.1,1.22464679914735E-16));
#22419=CARTESIAN_POINT('',(-1.,-0.1,-1.22464679914735E-16));
#22420=CARTESIAN_POINT('Origin',(0.,-0.1,0.));
#22421=CARTESIAN_POINT('',(0.,-0.625,-1.));
#22422=CARTESIAN_POINT('',(0.,-0.375,-1.));
#22423=CARTESIAN_POINT('Ctrl Pts',(-2.08166817117217E-17,-0.625,-1.));
#22424=CARTESIAN_POINT('Ctrl Pts',(0.0157128711428662,-0.625,-1.));
#22425=CARTESIAN_POINT('Ctrl Pts',(0.0324619190698279,-0.621856416896487,
-0.999591823858855));
#22426=CARTESIAN_POINT('Ctrl Pts',(0.0632545375991438,-0.609094573408246,
-0.998116453123232));
#22427=CARTESIAN_POINT('Ctrl Pts',(0.0772994769543644,-0.599477218342273,
-0.997070068816062));
#22428=CARTESIAN_POINT('Ctrl Pts',(0.0994773109804241,-0.577299384316213,
-0.995102104277285));
#22429=CARTESIAN_POINT('Ctrl Pts',(0.109094593469654,-0.563254485234654,
-0.994052129228928));
#22430=CARTESIAN_POINT('Ctrl Pts',(0.121856383722779,-0.532462003072536,
-0.99256853061881));
#22431=CARTESIAN_POINT('Ctrl Pts',(0.125,-0.515713002410637,-0.992156741649221));
#22432=CARTESIAN_POINT('Ctrl Pts',(0.125,-0.484286997589363,-0.992156741649221));
#22433=CARTESIAN_POINT('Ctrl Pts',(0.121856383722779,-0.467537996927464,
-0.99256853061881));
#22434=CARTESIAN_POINT('Ctrl Pts',(0.109094593469654,-0.436745514765346,
-0.994052129228928));
#22435=CARTESIAN_POINT('Ctrl Pts',(0.0994773109804241,-0.422700615683787,
-0.995102104277285));
#22436=CARTESIAN_POINT('Ctrl Pts',(0.0772994769543645,-0.400522781657728,
-0.997070068816062));
#22437=CARTESIAN_POINT('Ctrl Pts',(0.0632545375991439,-0.390905426591754,
-0.998116453123232));
#22438=CARTESIAN_POINT('Ctrl Pts',(0.032461919069828,-0.378143583103513,
-0.999591823858855));
#22439=CARTESIAN_POINT('Ctrl Pts',(0.0157128711428662,-0.375,-1.));
#22440=CARTESIAN_POINT('Ctrl Pts',(3.81639164714898E-17,-0.375,-1.));
#22441=CARTESIAN_POINT('',(-0.125,-0.5,-0.992156741649222));
#22442=CARTESIAN_POINT('Ctrl Pts',(4.5102810375397E-17,-0.375,-1.));
#22443=CARTESIAN_POINT('Ctrl Pts',(-0.0157128711428661,-0.375,-1.));
#22444=CARTESIAN_POINT('Ctrl Pts',(-0.0324619190698279,-0.378143583103513,
-0.999591823858855));
#22445=CARTESIAN_POINT('Ctrl Pts',(-0.0632545375991437,-0.390905426591754,
-0.998116453123232));
#22446=CARTESIAN_POINT('Ctrl Pts',(-0.0772994769543643,-0.400522781657727,
-0.997070068816062));
#22447=CARTESIAN_POINT('Ctrl Pts',(-0.099477310980424,-0.422700615683787,
-0.995102104277285));
#22448=CARTESIAN_POINT('Ctrl Pts',(-0.109094593469654,-0.436745514765346,
-0.994052129228928));
#22449=CARTESIAN_POINT('Ctrl Pts',(-0.121856383722779,-0.467537996927464,
-0.99256853061881));
#22450=CARTESIAN_POINT('Ctrl Pts',(-0.125,-0.484286997589363,-0.992156741649222));
#22451=CARTESIAN_POINT('Ctrl Pts',(-0.125,-0.5,-0.992156741649222));
#22452=CARTESIAN_POINT('Ctrl Pts',(-0.125,-0.5,-0.992156741649222));
#22453=CARTESIAN_POINT('Ctrl Pts',(-0.125,-0.515713002410637,-0.992156741649222));
#22454=CARTESIAN_POINT('Ctrl Pts',(-0.121856383722779,-0.532462003072536,
-0.99256853061881));
#22455=CARTESIAN_POINT('Ctrl Pts',(-0.109094593469654,-0.563254485234654,
-0.994052129228928));
#22456=CARTESIAN_POINT('Ctrl Pts',(-0.0994773109804241,-0.577299384316213,
-0.995102104277285));
#22457=CARTESIAN_POINT('Ctrl Pts',(-0.0772994769543644,-0.599477218342273,
-0.997070068816062));
#22458=CARTESIAN_POINT('Ctrl Pts',(-0.0632545375991439,-0.609094573408246,
-0.998116453123232));
#22459=CARTESIAN_POINT('Ctrl Pts',(-0.032461919069828,-0.621856416896487,
-0.999591823858855));
#22460=CARTESIAN_POINT('Ctrl Pts',(-0.0157128711428662,-0.625,-1.));
#22461=CARTESIAN_POINT('Ctrl Pts',(-1.38777878078145E-17,-0.625,-1.));
#22462=CARTESIAN_POINT('',(0.,-0.375,1.));
#22463=CARTESIAN_POINT('',(0.,-0.625,1.));
#22464=CARTESIAN_POINT('Ctrl Pts',(4.16333634234434E-17,-0.375,1.));
#22465=CARTESIAN_POINT('Ctrl Pts',(0.0157128711428662,-0.375,1.));
#22466=CARTESIAN_POINT('Ctrl Pts',(0.032461919069828,-0.378143583103513,
0.999591823858855));
#22467=CARTESIAN_POINT('Ctrl Pts',(0.0632545375991439,-0.390905426591754,
0.998116453123232));
#22468=CARTESIAN_POINT('Ctrl Pts',(0.0772994769543644,-0.400522781657728,
0.997070068816062));
#22469=CARTESIAN_POINT('Ctrl Pts',(0.0994773109804241,-0.422700615683787,
0.995102104277285));
#22470=CARTESIAN_POINT('Ctrl Pts',(0.109094593469654,-0.436745514765346,
0.994052129228928));
#22471=CARTESIAN_POINT('Ctrl Pts',(0.121856383722779,-0.467537996927464,
0.99256853061881));
#22472=CARTESIAN_POINT('Ctrl Pts',(0.125,-0.484286997589363,0.992156741649222));
#22473=CARTESIAN_POINT('Ctrl Pts',(0.125,-0.515713002410637,0.992156741649222));
#22474=CARTESIAN_POINT('Ctrl Pts',(0.121856383722779,-0.532462003072536,
0.99256853061881));
#22475=CARTESIAN_POINT('Ctrl Pts',(0.109094593469655,-0.563254485234654,
0.994052129228928));
#22476=CARTESIAN_POINT('Ctrl Pts',(0.0994773109804241,-0.577299384316213,
0.995102104277285));
#22477=CARTESIAN_POINT('Ctrl Pts',(0.0772994769543644,-0.599477218342273,
0.997070068816062));
#22478=CARTESIAN_POINT('Ctrl Pts',(0.0632545375991438,-0.609094573408246,
0.998116453123232));
#22479=CARTESIAN_POINT('Ctrl Pts',(0.0324619190698279,-0.621856416896487,
0.999591823858855));
#22480=CARTESIAN_POINT('Ctrl Pts',(0.0157128711428662,-0.625,1.));
#22481=CARTESIAN_POINT('Ctrl Pts',(-1.73472347597681E-17,-0.625,1.));
#22482=CARTESIAN_POINT('',(-0.125,-0.5,0.992156741649222));
#22483=CARTESIAN_POINT('Ctrl Pts',(-1.73472347597681E-17,-0.625,1.));
#22484=CARTESIAN_POINT('Ctrl Pts',(-0.0157128711428662,-0.625,1.));
#22485=CARTESIAN_POINT('Ctrl Pts',(-0.032461919069828,-0.621856416896487,
0.999591823858855));
#22486=CARTESIAN_POINT('Ctrl Pts',(-0.0632545375991439,-0.609094573408246,
0.998116453123232));
#22487=CARTESIAN_POINT('Ctrl Pts',(-0.0772994769543645,-0.599477218342273,
0.997070068816062));
#22488=CARTESIAN_POINT('Ctrl Pts',(-0.0994773109804241,-0.577299384316213,
0.995102104277285));
#22489=CARTESIAN_POINT('Ctrl Pts',(-0.109094593469654,-0.563254485234654,
0.994052129228928));
#22490=CARTESIAN_POINT('Ctrl Pts',(-0.121856383722779,-0.532462003072536,
0.99256853061881));
#22491=CARTESIAN_POINT('Ctrl Pts',(-0.125,-0.515713002410637,0.992156741649222));
#22492=CARTESIAN_POINT('Ctrl Pts',(-0.125,-0.5,0.992156741649222));
#22493=CARTESIAN_POINT('Ctrl Pts',(-0.125,-0.5,0.992156741649222));
#22494=CARTESIAN_POINT('Ctrl Pts',(-0.125,-0.484286997589363,0.992156741649222));
#22495=CARTESIAN_POINT('Ctrl Pts',(-0.121856383722779,-0.467537996927464,
0.99256853061881));
#22496=CARTESIAN_POINT('Ctrl Pts',(-0.109094593469654,-0.436745514765346,
0.994052129228928));
#22497=CARTESIAN_POINT('Ctrl Pts',(-0.099477310980424,-0.422700615683787,
0.995102104277285));
#22498=CARTESIAN_POINT('Ctrl Pts',(-0.0772994769543643,-0.400522781657727,
0.997070068816062));
#22499=CARTESIAN_POINT('Ctrl Pts',(-0.0632545375991438,-0.390905426591754,
0.998116453123232));
#22500=CARTESIAN_POINT('Ctrl Pts',(-0.0324619190698279,-0.378143583103513,
0.999591823858855));
#22501=CARTESIAN_POINT('Ctrl Pts',(-0.0157128711428661,-0.375,1.));
#22502=CARTESIAN_POINT('Ctrl Pts',(4.5102810375397E-17,-0.375,1.));
#22503=CARTESIAN_POINT('Origin',(0.,-0.5,0.));
#22504=CARTESIAN_POINT('',(-0.125,-0.5,-0.586834729715275));
#22505=CARTESIAN_POINT('',(-0.125,-0.5,0.));
#22506=CARTESIAN_POINT('',(0.125,-0.5,-0.586834729715275));
#22507=CARTESIAN_POINT('Ctrl Pts',(0.125,-0.5,-0.586834729715275));
#22508=CARTESIAN_POINT('Ctrl Pts',(0.125,-0.515745525063995,-0.586834729715275));
#22509=CARTESIAN_POINT('Ctrl Pts',(0.121843784097853,-0.532507913768158,
-0.587534197873268));
#22510=CARTESIAN_POINT('Ctrl Pts',(0.109073016834181,-0.563290995658393,
-0.590038488226116));
#22511=CARTESIAN_POINT('Ctrl Pts',(0.0994608796208942,-0.577315815675743,
-0.591804743154611));
#22512=CARTESIAN_POINT('Ctrl Pts',(0.077316548567853,-0.599460146728784,
-0.59510289473619));
#22513=CARTESIAN_POINT('Ctrl Pts',(0.0632914182239686,-0.609072857638709,
-0.596852269967858));
#22514=CARTESIAN_POINT('Ctrl Pts',(0.0325072544867633,-0.621844041497889,
-0.599317707212167));
#22515=CARTESIAN_POINT('Ctrl Pts',(0.0157444828659573,-0.625,-0.6));
#22516=CARTESIAN_POINT('Ctrl Pts',(-0.0157444828659572,-0.625,-0.6));
#22517=CARTESIAN_POINT('Ctrl Pts',(-0.0325072544867633,-0.621844041497889,
-0.599317707212167));
#22518=CARTESIAN_POINT('Ctrl Pts',(-0.0632914182239686,-0.609072857638709,
-0.596852269967858));
#22519=CARTESIAN_POINT('Ctrl Pts',(-0.077316548567853,-0.599460146728784,
-0.59510289473619));
#22520=CARTESIAN_POINT('Ctrl Pts',(-0.0994608796208941,-0.577315815675743,
-0.591804743154611));
#22521=CARTESIAN_POINT('Ctrl Pts',(-0.109073016834181,-0.563290995658393,
-0.590038488226116));
#22522=CARTESIAN_POINT('Ctrl Pts',(-0.121843784097853,-0.532507913768158,
-0.587534197873268));
#22523=CARTESIAN_POINT('Ctrl Pts',(-0.125,-0.515745525063995,-0.586834729715275));
#22524=CARTESIAN_POINT('Ctrl Pts',(-0.125,-0.5,-0.586834729715275));
#22525=CARTESIAN_POINT('Ctrl Pts',(-0.125,-0.5,-0.586834729715275));
#22526=CARTESIAN_POINT('Ctrl Pts',(-0.125,-0.484254474936005,-0.586834729715275));
#22527=CARTESIAN_POINT('Ctrl Pts',(-0.121843784097853,-0.467492086231842,
-0.587534197873268));
#22528=CARTESIAN_POINT('Ctrl Pts',(-0.109073016834181,-0.436709004341607,
-0.590038488226116));
#22529=CARTESIAN_POINT('Ctrl Pts',(-0.0994608796208942,-0.422684184324257,
-0.591804743154611));
#22530=CARTESIAN_POINT('Ctrl Pts',(-0.077316548567853,-0.400539853271216,
-0.59510289473619));
#22531=CARTESIAN_POINT('Ctrl Pts',(-0.0632914182239687,-0.39092714236129,
-0.596852269967858));
#22532=CARTESIAN_POINT('Ctrl Pts',(-0.0325072544867634,-0.378155958502111,
-0.599317707212167));
#22533=CARTESIAN_POINT('Ctrl Pts',(-0.0157444828659573,-0.375,-0.6));
#22534=CARTESIAN_POINT('Ctrl Pts',(0.0157444828659572,-0.375,-0.6));
#22535=CARTESIAN_POINT('Ctrl Pts',(0.0325072544867634,-0.378155958502111,
-0.599317707212167));
#22536=CARTESIAN_POINT('Ctrl Pts',(0.0632914182239686,-0.390927142361291,
-0.596852269967858));
#22537=CARTESIAN_POINT('Ctrl Pts',(0.077316548567853,-0.400539853271216,
-0.59510289473619));
#22538=CARTESIAN_POINT('Ctrl Pts',(0.0994608796208941,-0.422684184324257,
-0.591804743154611));
#22539=CARTESIAN_POINT('Ctrl Pts',(0.109073016834181,-0.436709004341607,
-0.590038488226116));
#22540=CARTESIAN_POINT('Ctrl Pts',(0.121843784097853,-0.467492086231842,
-0.587534197873268));
#22541=CARTESIAN_POINT('Ctrl Pts',(0.125,-0.484254474936005,-0.586834729715275));
#22542=CARTESIAN_POINT('Ctrl Pts',(0.125,-0.5,-0.586834729715275));
#22543=CARTESIAN_POINT('Origin',(0.,-0.5,0.));
#22544=CARTESIAN_POINT('',(0.125,-0.5,0.586834729715275));
#22545=CARTESIAN_POINT('',(-0.125,-0.5,0.586834729715275));
#22546=CARTESIAN_POINT('Ctrl Pts',(0.125,-0.5,0.586834729715275));
#22547=CARTESIAN_POINT('Ctrl Pts',(0.125,-0.484254474936005,0.586834729715275));
#22548=CARTESIAN_POINT('Ctrl Pts',(0.121843784097853,-0.467492086231842,
0.587534197873268));
#22549=CARTESIAN_POINT('Ctrl Pts',(0.109073016834181,-0.436709004341607,
0.590038488226116));
#22550=CARTESIAN_POINT('Ctrl Pts',(0.0994608796208941,-0.422684184324257,
0.591804743154611));
#22551=CARTESIAN_POINT('Ctrl Pts',(0.077316548567853,-0.400539853271216,
0.59510289473619));
#22552=CARTESIAN_POINT('Ctrl Pts',(0.0632914182239686,-0.390927142361291,
0.596852269967858));
#22553=CARTESIAN_POINT('Ctrl Pts',(0.0325072544867634,-0.378155958502111,
0.599317707212167));
#22554=CARTESIAN_POINT('Ctrl Pts',(0.0157444828659572,-0.375,0.6));
#22555=CARTESIAN_POINT('Ctrl Pts',(-0.0157444828659573,-0.375,0.6));
#22556=CARTESIAN_POINT('Ctrl Pts',(-0.0325072544867634,-0.378155958502111,
0.599317707212167));
#22557=CARTESIAN_POINT('Ctrl Pts',(-0.0632914182239687,-0.390927142361291,
0.596852269967858));
#22558=CARTESIAN_POINT('Ctrl Pts',(-0.077316548567853,-0.400539853271216,
0.59510289473619));
#22559=CARTESIAN_POINT('Ctrl Pts',(-0.0994608796208942,-0.422684184324257,
0.591804743154611));
#22560=CARTESIAN_POINT('Ctrl Pts',(-0.109073016834181,-0.436709004341607,
0.590038488226116));
#22561=CARTESIAN_POINT('Ctrl Pts',(-0.121843784097853,-0.467492086231842,
0.587534197873268));
#22562=CARTESIAN_POINT('Ctrl Pts',(-0.125,-0.484254474936005,0.586834729715275));
#22563=CARTESIAN_POINT('Ctrl Pts',(-0.125,-0.5,0.586834729715275));
#22564=CARTESIAN_POINT('Ctrl Pts',(-0.125,-0.5,0.586834729715275));
#22565=CARTESIAN_POINT('Ctrl Pts',(-0.125,-0.515745525063995,0.586834729715275));
#22566=CARTESIAN_POINT('Ctrl Pts',(-0.121843784097853,-0.532507913768158,
0.587534197873268));
#22567=CARTESIAN_POINT('Ctrl Pts',(-0.109073016834181,-0.563290995658393,
0.590038488226116));
#22568=CARTESIAN_POINT('Ctrl Pts',(-0.0994608796208941,-0.577315815675743,
0.591804743154611));
#22569=CARTESIAN_POINT('Ctrl Pts',(-0.077316548567853,-0.599460146728784,
0.59510289473619));
#22570=CARTESIAN_POINT('Ctrl Pts',(-0.0632914182239687,-0.609072857638709,
0.596852269967858));
#22571=CARTESIAN_POINT('Ctrl Pts',(-0.0325072544867635,-0.621844041497889,
0.599317707212167));
#22572=CARTESIAN_POINT('Ctrl Pts',(-0.0157444828659572,-0.625,0.6));
#22573=CARTESIAN_POINT('Ctrl Pts',(0.0157444828659572,-0.625,0.6));
#22574=CARTESIAN_POINT('Ctrl Pts',(0.0325072544867633,-0.621844041497889,
0.599317707212167));
#22575=CARTESIAN_POINT('Ctrl Pts',(0.0632914182239686,-0.609072857638709,
0.596852269967858));
#22576=CARTESIAN_POINT('Ctrl Pts',(0.077316548567853,-0.599460146728784,
0.59510289473619));
#22577=CARTESIAN_POINT('Ctrl Pts',(0.0994608796208942,-0.577315815675743,
0.591804743154611));
#22578=CARTESIAN_POINT('Ctrl Pts',(0.109073016834181,-0.563290995658393,
0.590038488226116));
#22579=CARTESIAN_POINT('Ctrl Pts',(0.121843784097853,-0.532507913768158,
0.587534197873268));
#22580=CARTESIAN_POINT('Ctrl Pts',(0.125,-0.515745525063995,0.586834729715275));
#22581=CARTESIAN_POINT('Ctrl Pts',(0.125,-0.5,0.586834729715275));
#22582=CARTESIAN_POINT('',(-0.125,-0.5,0.));
#22583=CARTESIAN_POINT('Origin',(0.,0.,0.));
#22584=CARTESIAN_POINT('',(-0.6,-0.9,7.34788079488412E-17));
#22585=CARTESIAN_POINT('Origin',(0.,-0.9,0.));
#22586=CARTESIAN_POINT('',(-0.6,0.,7.34788079488412E-17));
#22587=CARTESIAN_POINT('',(-0.6,0.85,-7.34788079488412E-17));
#22588=CARTESIAN_POINT('',(-0.6,0.,7.34788079488412E-17));
#22589=CARTESIAN_POINT('Origin',(0.,0.85,0.));
#22590=CARTESIAN_POINT('Origin',(0.,-0.9,0.));
#22591=CARTESIAN_POINT('Origin',(0.,0.,0.));
#22592=CARTESIAN_POINT('',(-1.4,0.,1.71450551880629E-16));
#22593=CARTESIAN_POINT('Origin',(0.,0.,0.));
#22594=CARTESIAN_POINT('',(1.23958209161204,0.,0.143317017690053));
#22595=CARTESIAN_POINT('',(1.22320001975977,0.,0.246749348660852));
#22596=CARTESIAN_POINT('Origin',(1.21321664662686,0.,0.192154639568406));
#22597=CARTESIAN_POINT('',(1.20190105810224,0.,0.335465908756113));
#22598=CARTESIAN_POINT('Origin',(0.,0.,0.));
#22599=CARTESIAN_POINT('',(1.16954029537568,0.,0.435062095450087));
#22600=CARTESIAN_POINT('Origin',(1.1682203282434,0.,0.379577794185952));
#22601=CARTESIAN_POINT('',(1.13462523166105,0.,0.519354515801077));
#22602=CARTESIAN_POINT('Origin',(0.,0.,0.));
#22603=CARTESIAN_POINT('',(1.08708260743774,0.,0.612662169561029));
#22604=CARTESIAN_POINT('Origin',(1.0944585482776,0.,0.557654483764164));
#22605=CARTESIAN_POINT('',(1.0394111664111,0.,0.690454891028201));
#22606=CARTESIAN_POINT('Origin',(0.,0.,0.));
#22607=CARTESIAN_POINT('',(0.977857337884349,0.,0.775176467748211));
#22608=CARTESIAN_POINT('Origin',(0.993747566553533,0.,0.72199986920298));
#22609=CARTESIAN_POINT('',(0.918603348636233,0.,0.844553975349804));
#22610=CARTESIAN_POINT('Origin',(0.,0.,0.));
#22611=CARTESIAN_POINT('',(0.844553975349804,0.,0.918603348636233));
#22612=CARTESIAN_POINT('Origin',(0.86856722168183,0.,0.86856722168183));
#22613=CARTESIAN_POINT('',(0.775176467748211,0.,0.977857337884349));
#22614=CARTESIAN_POINT('Origin',(0.,0.,0.));
#22615=CARTESIAN_POINT('',(0.690454891028201,0.,1.0394111664111));
#22616=CARTESIAN_POINT('Origin',(0.721999869202979,0.,0.993747566553533));
#22617=CARTESIAN_POINT('',(0.612662169561028,0.,1.08708260743774));
#22618=CARTESIAN_POINT('Origin',(0.,0.,0.));
#22619=CARTESIAN_POINT('',(0.519354515801077,0.,1.13462523166105));
#22620=CARTESIAN_POINT('Origin',(0.557654483764164,0.,1.0944585482776));
#22621=CARTESIAN_POINT('',(0.435062095450087,0.,1.16954029537568));
#22622=CARTESIAN_POINT('Origin',(0.,0.,0.));
#22623=CARTESIAN_POINT('',(0.335465908756113,0.,1.20190105810224));
#22624=CARTESIAN_POINT('Origin',(0.379577794185951,0.,1.1682203282434));
#22625=CARTESIAN_POINT('',(0.246749348660851,0.,1.22320001975977));
#22626=CARTESIAN_POINT('Origin',(0.,0.,0.));
#22627=CARTESIAN_POINT('',(0.143317017690053,0.,1.23958209161204));
#22628=CARTESIAN_POINT('Origin',(0.192154639568406,0.,1.21321664662686));
#22629=CARTESIAN_POINT('',(0.0523608139934478,0.,1.24674050008925));
#22630=CARTESIAN_POINT('Origin',(0.,0.,0.));
#22631=CARTESIAN_POINT('',(-0.0523608139934483,0.,1.24674050008925));
#22632=CARTESIAN_POINT('Origin',(-2.25642313758905E-16,0.,1.22833954473516));
#22633=CARTESIAN_POINT('',(-0.143317017690053,0.,1.23958209161204));
#22634=CARTESIAN_POINT('Origin',(0.,0.,0.));
#22635=CARTESIAN_POINT('',(-0.246749348660852,0.,1.22320001975977));
#22636=CARTESIAN_POINT('Origin',(-0.192154639568406,0.,1.21321664662686));
#22637=CARTESIAN_POINT('',(-0.335465908756113,0.,1.20190105810224));
#22638=CARTESIAN_POINT('Origin',(0.,0.,0.));
#22639=CARTESIAN_POINT('',(-0.435062095450087,0.,1.16954029537568));
#22640=CARTESIAN_POINT('Origin',(-0.379577794185951,0.,1.1682203282434));
#22641=CARTESIAN_POINT('',(-0.519354515801077,0.,1.13462523166105));
#22642=CARTESIAN_POINT('Origin',(0.,0.,0.));
#22643=CARTESIAN_POINT('',(-0.612662169561029,0.,1.08708260743774));
#22644=CARTESIAN_POINT('Origin',(-0.557654483764164,0.,1.0944585482776));
#22645=CARTESIAN_POINT('',(-0.690454891028201,0.,1.0394111664111));
#22646=CARTESIAN_POINT('Origin',(0.,0.,0.));
#22647=CARTESIAN_POINT('',(-0.775176467748211,0.,0.977857337884349));
#22648=CARTESIAN_POINT('Origin',(-0.721999869202979,0.,0.993747566553533));
#22649=CARTESIAN_POINT('',(-0.844553975349804,0.,0.918603348636233));
#22650=CARTESIAN_POINT('Origin',(0.,0.,0.));
#22651=CARTESIAN_POINT('',(-0.918603348636233,0.,0.844553975349804));
#22652=CARTESIAN_POINT('Origin',(-0.86856722168183,0.,0.86856722168183));
#22653=CARTESIAN_POINT('',(-0.977857337884348,0.,0.775176467748211));
#22654=CARTESIAN_POINT('Origin',(0.,0.,0.));
#22655=CARTESIAN_POINT('',(-1.0394111664111,0.,0.690454891028201));
#22656=CARTESIAN_POINT('Origin',(-0.993747566553533,0.,0.721999869202979));
#22657=CARTESIAN_POINT('',(-1.08708260743774,0.,0.612662169561028));
#22658=CARTESIAN_POINT('Origin',(0.,0.,0.));
#22659=CARTESIAN_POINT('',(-1.13462523166105,0.,0.519354515801077));
#22660=CARTESIAN_POINT('Origin',(-1.0944585482776,0.,0.557654483764164));
#22661=CARTESIAN_POINT('',(-1.16954029537568,0.,0.435062095450087));
#22662=CARTESIAN_POINT('Origin',(0.,0.,0.));
#22663=CARTESIAN_POINT('',(-1.20190105810224,0.,0.335465908756113));
#22664=CARTESIAN_POINT('Origin',(-1.1682203282434,0.,0.379577794185951));
#22665=CARTESIAN_POINT('',(-1.22320001975977,0.,0.246749348660851));
#22666=CARTESIAN_POINT('Origin',(0.,0.,0.));
#22667=CARTESIAN_POINT('',(-1.23958209161204,0.,0.143317017690053));
#22668=CARTESIAN_POINT('Origin',(-1.21321664662686,0.,0.192154639568406));
#22669=CARTESIAN_POINT('',(-1.24674050008925,0.,0.0523608139934479));
#22670=CARTESIAN_POINT('Origin',(0.,0.,0.));
#22671=CARTESIAN_POINT('',(-1.24674050008925,0.,-0.0523608139934482));
#22672=CARTESIAN_POINT('Origin',(-1.22833954473516,0.,-1.50428209172603E-16));
#22673=CARTESIAN_POINT('',(-1.23958209161204,0.,-0.143317017690053));
#22674=CARTESIAN_POINT('Origin',(0.,0.,0.));
#22675=CARTESIAN_POINT('',(-1.22320001975977,0.,-0.246749348660852));
#22676=CARTESIAN_POINT('Origin',(-1.21321664662686,0.,-0.192154639568406));
#22677=CARTESIAN_POINT('',(-1.20190105810224,0.,-0.335465908756113));
#22678=CARTESIAN_POINT('Origin',(0.,0.,0.));
#22679=CARTESIAN_POINT('',(-1.16954029537568,0.,-0.435062095450087));
#22680=CARTESIAN_POINT('Origin',(-1.1682203282434,0.,-0.379577794185951));
#22681=CARTESIAN_POINT('',(-1.13462523166105,0.,-0.519354515801077));
#22682=CARTESIAN_POINT('Origin',(0.,0.,0.));
#22683=CARTESIAN_POINT('',(-1.08708260743774,0.,-0.612662169561029));
#22684=CARTESIAN_POINT('Origin',(-1.0944585482776,0.,-0.557654483764164));
#22685=CARTESIAN_POINT('',(-1.0394111664111,0.,-0.690454891028201));
#22686=CARTESIAN_POINT('Origin',(0.,0.,0.));
#22687=CARTESIAN_POINT('',(-0.977857337884349,0.,-0.775176467748211));
#22688=CARTESIAN_POINT('Origin',(-0.993747566553533,0.,-0.721999869202979));
#22689=CARTESIAN_POINT('',(-0.918603348636233,0.,-0.844553975349804));
#22690=CARTESIAN_POINT('Origin',(0.,0.,0.));
#22691=CARTESIAN_POINT('',(-0.844553975349804,0.,-0.918603348636233));
#22692=CARTESIAN_POINT('Origin',(-0.86856722168183,0.,-0.86856722168183));
#22693=CARTESIAN_POINT('',(-0.775176467748211,0.,-0.977857337884348));
#22694=CARTESIAN_POINT('Origin',(0.,0.,0.));
#22695=CARTESIAN_POINT('',(-0.690454891028201,0.,-1.0394111664111));
#22696=CARTESIAN_POINT('Origin',(-0.721999869202979,0.,-0.993747566553533));
#22697=CARTESIAN_POINT('',(-0.612662169561028,0.,-1.08708260743774));
#22698=CARTESIAN_POINT('Origin',(0.,0.,0.));
#22699=CARTESIAN_POINT('',(-0.519354515801077,0.,-1.13462523166105));
#22700=CARTESIAN_POINT('Origin',(-0.557654483764164,0.,-1.0944585482776));
#22701=CARTESIAN_POINT('',(-0.435062095450087,0.,-1.16954029537568));
#22702=CARTESIAN_POINT('Origin',(0.,0.,0.));
#22703=CARTESIAN_POINT('',(-0.335465908756113,0.,-1.20190105810224));
#22704=CARTESIAN_POINT('Origin',(-0.379577794185951,0.,-1.1682203282434));
#22705=CARTESIAN_POINT('',(-0.246749348660852,0.,-1.22320001975977));
#22706=CARTESIAN_POINT('Origin',(0.,0.,0.));
#22707=CARTESIAN_POINT('',(-0.143317017690053,0.,-1.23958209161204));
#22708=CARTESIAN_POINT('Origin',(-0.192154639568406,0.,-1.21321664662686));
#22709=CARTESIAN_POINT('',(-0.0523608139934479,0.,-1.24674050008925));
#22710=CARTESIAN_POINT('Origin',(0.,0.,0.));
#22711=CARTESIAN_POINT('',(0.0523608139934481,0.,-1.24674050008925));
#22712=CARTESIAN_POINT('Origin',(7.52141045863017E-17,0.,-1.22833954473516));
#22713=CARTESIAN_POINT('',(0.143317017690053,0.,-1.23958209161204));
#22714=CARTESIAN_POINT('Origin',(0.,0.,0.));
#22715=CARTESIAN_POINT('',(0.246749348660852,0.,-1.22320001975977));
#22716=CARTESIAN_POINT('Origin',(0.192154639568406,0.,-1.21321664662686));
#22717=CARTESIAN_POINT('',(0.335465908756113,0.,-1.20190105810224));
#22718=CARTESIAN_POINT('Origin',(0.,0.,0.));
#22719=CARTESIAN_POINT('',(0.435062095450087,0.,-1.16954029537568));
#22720=CARTESIAN_POINT('Origin',(0.379577794185951,0.,-1.1682203282434));
#22721=CARTESIAN_POINT('',(0.519354515801077,0.,-1.13462523166105));
#22722=CARTESIAN_POINT('Origin',(0.,0.,0.));
#22723=CARTESIAN_POINT('',(0.612662169561028,0.,-1.08708260743774));
#22724=CARTESIAN_POINT('Origin',(0.557654483764164,0.,-1.0944585482776));
#22725=CARTESIAN_POINT('',(0.690454891028201,0.,-1.0394111664111));
#22726=CARTESIAN_POINT('Origin',(0.,0.,0.));
#22727=CARTESIAN_POINT('',(0.775176467748211,0.,-0.977857337884349));
#22728=CARTESIAN_POINT('Origin',(0.721999869202979,0.,-0.993747566553533));
#22729=CARTESIAN_POINT('',(0.844553975349804,0.,-0.918603348636233));
#22730=CARTESIAN_POINT('Origin',(0.,0.,0.));
#22731=CARTESIAN_POINT('',(0.918603348636233,0.,-0.844553975349804));
#22732=CARTESIAN_POINT('Origin',(0.86856722168183,0.,-0.86856722168183));
#22733=CARTESIAN_POINT('',(0.977857337884349,0.,-0.775176467748211));
#22734=CARTESIAN_POINT('Origin',(0.,0.,0.));
#22735=CARTESIAN_POINT('',(1.0394111664111,0.,-0.690454891028201));
#22736=CARTESIAN_POINT('Origin',(0.993747566553533,0.,-0.721999869202979));
#22737=CARTESIAN_POINT('',(1.08708260743774,0.,-0.612662169561028));
#22738=CARTESIAN_POINT('Origin',(0.,0.,0.));
#22739=CARTESIAN_POINT('',(1.13462523166105,0.,-0.519354515801077));
#22740=CARTESIAN_POINT('Origin',(1.0944585482776,0.,-0.557654483764164));
#22741=CARTESIAN_POINT('',(1.16954029537568,0.,-0.43506209545009));
#22742=CARTESIAN_POINT('Origin',(0.,0.,0.));
#22743=CARTESIAN_POINT('',(1.20190105810224,0.,-0.33546590875611));
#22744=CARTESIAN_POINT('Origin',(1.1682203282434,0.,-0.379577794185951));
#22745=CARTESIAN_POINT('',(1.22320001975977,0.,-0.246749348660852));
#22746=CARTESIAN_POINT('Origin',(0.,0.,0.));
#22747=CARTESIAN_POINT('',(1.23958209161204,0.,-0.143317017690053));
#22748=CARTESIAN_POINT('Origin',(1.21321664662686,0.,-0.192154639568406));
#22749=CARTESIAN_POINT('',(1.24674050008925,0.,-0.052360813993451));
#22750=CARTESIAN_POINT('Origin',(0.,0.,0.));
#22751=CARTESIAN_POINT('',(1.24674050008925,0.,0.052360813993451));
#22752=CARTESIAN_POINT('Origin',(1.22833954473516,0.,0.));
#22753=CARTESIAN_POINT('Origin',(0.,0.,0.));
#22754=CARTESIAN_POINT('Origin',(0.,0.,0.));
#22755=CARTESIAN_POINT('',(-1.4,-0.1,1.71450551880629E-16));
#22756=CARTESIAN_POINT('Origin',(0.,-0.1,0.));
#22757=CARTESIAN_POINT('',(-1.4,0.,-1.71450551880629E-16));
#22758=CARTESIAN_POINT('Origin',(0.,-0.1,0.));
#22759=CARTESIAN_POINT('Origin',(0.,0.75,0.));
#22760=CARTESIAN_POINT('',(-1.4,0.75,1.71450551880629E-16));
#22761=CARTESIAN_POINT('Origin',(0.,0.75,0.));
#22762=CARTESIAN_POINT('',(1.22320001975977,0.75,0.246749348660852));
#22763=CARTESIAN_POINT('',(1.23958209161204,0.75,0.143317017690053));
#22764=CARTESIAN_POINT('Origin',(1.21321664662686,0.75,0.192154639568406));
#22765=CARTESIAN_POINT('',(1.24674050008925,0.75,0.052360813993448));
#22766=CARTESIAN_POINT('Origin',(0.,0.75,0.));
#22767=CARTESIAN_POINT('',(1.24674050008925,0.75,-0.052360813993448));
#22768=CARTESIAN_POINT('Origin',(1.22833954473516,0.75,0.));
#22769=CARTESIAN_POINT('',(1.23958209161204,0.75,-0.143317017690053));
#22770=CARTESIAN_POINT('Origin',(0.,0.75,0.));
#22771=CARTESIAN_POINT('',(1.22320001975977,0.75,-0.246749348660852));
#22772=CARTESIAN_POINT('Origin',(1.21321664662686,0.75,-0.192154639568406));
#22773=CARTESIAN_POINT('',(1.20190105810224,0.75,-0.335465908756113));
#22774=CARTESIAN_POINT('Origin',(0.,0.75,0.));
#22775=CARTESIAN_POINT('',(1.16954029537568,0.75,-0.435062095450087));
#22776=CARTESIAN_POINT('Origin',(1.1682203282434,0.75,-0.379577794185951));
#22777=CARTESIAN_POINT('',(1.13462523166105,0.75,-0.519354515801077));
#22778=CARTESIAN_POINT('Origin',(0.,0.75,0.));
#22779=CARTESIAN_POINT('',(1.08708260743774,0.75,-0.612662169561028));
#22780=CARTESIAN_POINT('Origin',(1.0944585482776,0.75,-0.557654483764164));
#22781=CARTESIAN_POINT('',(1.0394111664111,0.75,-0.690454891028201));
#22782=CARTESIAN_POINT('Origin',(0.,0.75,0.));
#22783=CARTESIAN_POINT('',(0.977857337884349,0.75,-0.775176467748211));
#22784=CARTESIAN_POINT('Origin',(0.993747566553533,0.75,-0.721999869202979));
#22785=CARTESIAN_POINT('',(0.918603348636233,0.75,-0.844553975349804));
#22786=CARTESIAN_POINT('Origin',(0.,0.75,0.));
#22787=CARTESIAN_POINT('',(0.844553975349804,0.75,-0.918603348636233));
#22788=CARTESIAN_POINT('Origin',(0.86856722168183,0.75,-0.86856722168183));
#22789=CARTESIAN_POINT('',(0.775176467748211,0.75,-0.977857337884349));
#22790=CARTESIAN_POINT('Origin',(0.,0.75,0.));
#22791=CARTESIAN_POINT('',(0.690454891028201,0.75,-1.0394111664111));
#22792=CARTESIAN_POINT('Origin',(0.721999869202979,0.75,-0.993747566553533));
#22793=CARTESIAN_POINT('',(0.612662169561028,0.75,-1.08708260743774));
#22794=CARTESIAN_POINT('Origin',(0.,0.75,0.));
#22795=CARTESIAN_POINT('',(0.519354515801077,0.75,-1.13462523166105));
#22796=CARTESIAN_POINT('Origin',(0.557654483764164,0.75,-1.0944585482776));
#22797=CARTESIAN_POINT('',(0.435062095450087,0.75,-1.16954029537568));
#22798=CARTESIAN_POINT('Origin',(0.,0.75,0.));
#22799=CARTESIAN_POINT('',(0.335465908756113,0.75,-1.20190105810224));
#22800=CARTESIAN_POINT('Origin',(0.379577794185951,0.75,-1.1682203282434));
#22801=CARTESIAN_POINT('',(0.246749348660852,0.75,-1.22320001975977));
#22802=CARTESIAN_POINT('Origin',(0.,0.75,0.));
#22803=CARTESIAN_POINT('',(0.143317017690053,0.75,-1.23958209161204));
#22804=CARTESIAN_POINT('Origin',(0.192154639568406,0.75,-1.21321664662686));
#22805=CARTESIAN_POINT('',(0.0523608139934481,0.75,-1.24674050008925));
#22806=CARTESIAN_POINT('Origin',(0.,0.75,0.));
#22807=CARTESIAN_POINT('',(-0.0523608139934479,0.75,-1.24674050008925));
#22808=CARTESIAN_POINT('Origin',(7.52141045863017E-17,0.75,-1.22833954473516));
#22809=CARTESIAN_POINT('',(-0.143317017690053,0.75,-1.23958209161204));
#22810=CARTESIAN_POINT('Origin',(0.,0.75,0.));
#22811=CARTESIAN_POINT('',(-0.246749348660852,0.75,-1.22320001975977));
#22812=CARTESIAN_POINT('Origin',(-0.192154639568406,0.75,-1.21321664662686));
#22813=CARTESIAN_POINT('',(-0.335465908756113,0.75,-1.20190105810224));
#22814=CARTESIAN_POINT('Origin',(0.,0.75,0.));
#22815=CARTESIAN_POINT('',(-0.435062095450087,0.75,-1.16954029537568));
#22816=CARTESIAN_POINT('Origin',(-0.379577794185951,0.75,-1.1682203282434));
#22817=CARTESIAN_POINT('',(-0.519354515801077,0.75,-1.13462523166105));
#22818=CARTESIAN_POINT('Origin',(0.,0.75,0.));
#22819=CARTESIAN_POINT('',(-0.612662169561028,0.75,-1.08708260743774));
#22820=CARTESIAN_POINT('Origin',(-0.557654483764164,0.75,-1.0944585482776));
#22821=CARTESIAN_POINT('',(-0.690454891028201,0.75,-1.0394111664111));
#22822=CARTESIAN_POINT('Origin',(0.,0.75,0.));
#22823=CARTESIAN_POINT('',(-0.775176467748211,0.75,-0.977857337884348));
#22824=CARTESIAN_POINT('Origin',(-0.721999869202979,0.75,-0.993747566553533));
#22825=CARTESIAN_POINT('',(-0.844553975349804,0.75,-0.918603348636233));
#22826=CARTESIAN_POINT('Origin',(0.,0.75,0.));
#22827=CARTESIAN_POINT('',(-0.918603348636233,0.75,-0.844553975349804));
#22828=CARTESIAN_POINT('Origin',(-0.86856722168183,0.75,-0.86856722168183));
#22829=CARTESIAN_POINT('',(-0.977857337884349,0.75,-0.775176467748211));
#22830=CARTESIAN_POINT('Origin',(0.,0.75,0.));
#22831=CARTESIAN_POINT('',(-1.0394111664111,0.75,-0.690454891028201));
#22832=CARTESIAN_POINT('Origin',(-0.993747566553533,0.75,-0.721999869202979));
#22833=CARTESIAN_POINT('',(-1.08708260743774,0.75,-0.612662169561029));
#22834=CARTESIAN_POINT('Origin',(0.,0.75,0.));
#22835=CARTESIAN_POINT('',(-1.13462523166105,0.75,-0.519354515801077));
#22836=CARTESIAN_POINT('Origin',(-1.0944585482776,0.75,-0.557654483764164));
#22837=CARTESIAN_POINT('',(-1.16954029537568,0.75,-0.435062095450087));
#22838=CARTESIAN_POINT('Origin',(0.,0.75,0.));
#22839=CARTESIAN_POINT('',(-1.20190105810224,0.75,-0.335465908756113));
#22840=CARTESIAN_POINT('Origin',(-1.1682203282434,0.75,-0.379577794185951));
#22841=CARTESIAN_POINT('',(-1.22320001975977,0.75,-0.246749348660852));
#22842=CARTESIAN_POINT('Origin',(0.,0.75,0.));
#22843=CARTESIAN_POINT('',(-1.23958209161204,0.75,-0.143317017690053));
#22844=CARTESIAN_POINT('Origin',(-1.21321664662686,0.75,-0.192154639568406));
#22845=CARTESIAN_POINT('',(-1.24674050008925,0.75,-0.0523608139934482));
#22846=CARTESIAN_POINT('Origin',(0.,0.75,0.));
#22847=CARTESIAN_POINT('',(-1.24674050008925,0.75,0.0523608139934479));
#22848=CARTESIAN_POINT('Origin',(-1.22833954473516,0.75,-1.50428209172603E-16));
#22849=CARTESIAN_POINT('',(-1.23958209161204,0.75,0.143317017690053));
#22850=CARTESIAN_POINT('Origin',(0.,0.75,0.));
#22851=CARTESIAN_POINT('',(-1.22320001975977,0.75,0.246749348660851));
#22852=CARTESIAN_POINT('Origin',(-1.21321664662686,0.75,0.192154639568406));
#22853=CARTESIAN_POINT('',(-1.20190105810224,0.75,0.335465908756113));
#22854=CARTESIAN_POINT('Origin',(0.,0.75,0.));
#22855=CARTESIAN_POINT('',(-1.16954029537568,0.75,0.435062095450087));
#22856=CARTESIAN_POINT('Origin',(-1.1682203282434,0.75,0.379577794185951));
#22857=CARTESIAN_POINT('',(-1.13462523166105,0.75,0.519354515801077));
#22858=CARTESIAN_POINT('Origin',(0.,0.75,0.));
#22859=CARTESIAN_POINT('',(-1.08708260743774,0.75,0.612662169561028));
#22860=CARTESIAN_POINT('Origin',(-1.0944585482776,0.75,0.557654483764164));
#22861=CARTESIAN_POINT('',(-1.0394111664111,0.75,0.690454891028201));
#22862=CARTESIAN_POINT('Origin',(0.,0.75,0.));
#22863=CARTESIAN_POINT('',(-0.977857337884348,0.75,0.775176467748211));
#22864=CARTESIAN_POINT('Origin',(-0.993747566553533,0.75,0.721999869202979));
#22865=CARTESIAN_POINT('',(-0.918603348636233,0.75,0.844553975349804));
#22866=CARTESIAN_POINT('Origin',(0.,0.75,0.));
#22867=CARTESIAN_POINT('',(-0.844553975349804,0.75,0.918603348636233));
#22868=CARTESIAN_POINT('Origin',(-0.86856722168183,0.75,0.86856722168183));
#22869=CARTESIAN_POINT('',(-0.775176467748211,0.75,0.977857337884349));
#22870=CARTESIAN_POINT('Origin',(0.,0.75,0.));
#22871=CARTESIAN_POINT('',(-0.690454891028201,0.75,1.0394111664111));
#22872=CARTESIAN_POINT('Origin',(-0.721999869202979,0.75,0.993747566553533));
#22873=CARTESIAN_POINT('',(-0.612662169561029,0.75,1.08708260743774));
#22874=CARTESIAN_POINT('Origin',(0.,0.75,0.));
#22875=CARTESIAN_POINT('',(-0.519354515801077,0.75,1.13462523166105));
#22876=CARTESIAN_POINT('Origin',(-0.557654483764164,0.75,1.0944585482776));
#22877=CARTESIAN_POINT('',(-0.435062095450087,0.75,1.16954029537568));
#22878=CARTESIAN_POINT('Origin',(0.,0.75,0.));
#22879=CARTESIAN_POINT('',(-0.335465908756113,0.75,1.20190105810224));
#22880=CARTESIAN_POINT('Origin',(-0.379577794185951,0.75,1.1682203282434));
#22881=CARTESIAN_POINT('',(-0.246749348660852,0.75,1.22320001975977));
#22882=CARTESIAN_POINT('Origin',(0.,0.75,0.));
#22883=CARTESIAN_POINT('',(-0.143317017690053,0.75,1.23958209161204));
#22884=CARTESIAN_POINT('Origin',(-0.192154639568406,0.75,1.21321664662686));
#22885=CARTESIAN_POINT('',(-0.0523608139934483,0.75,1.24674050008925));
#22886=CARTESIAN_POINT('Origin',(0.,0.75,0.));
#22887=CARTESIAN_POINT('',(0.0523608139934478,0.75,1.24674050008925));
#22888=CARTESIAN_POINT('Origin',(-2.25642313758905E-16,0.75,1.22833954473516));
#22889=CARTESIAN_POINT('',(0.143317017690053,0.75,1.23958209161204));
#22890=CARTESIAN_POINT('Origin',(0.,0.75,0.));
#22891=CARTESIAN_POINT('',(0.246749348660851,0.75,1.22320001975977));
#22892=CARTESIAN_POINT('Origin',(0.192154639568406,0.75,1.21321664662686));
#22893=CARTESIAN_POINT('',(0.335465908756113,0.75,1.20190105810224));
#22894=CARTESIAN_POINT('Origin',(0.,0.75,0.));
#22895=CARTESIAN_POINT('',(0.435062095450087,0.75,1.16954029537568));
#22896=CARTESIAN_POINT('Origin',(0.379577794185951,0.75,1.1682203282434));
#22897=CARTESIAN_POINT('',(0.519354515801077,0.75,1.13462523166105));
#22898=CARTESIAN_POINT('Origin',(0.,0.75,0.));
#22899=CARTESIAN_POINT('',(0.612662169561028,0.75,1.08708260743774));
#22900=CARTESIAN_POINT('Origin',(0.557654483764164,0.75,1.0944585482776));
#22901=CARTESIAN_POINT('',(0.690454891028201,0.75,1.0394111664111));
#22902=CARTESIAN_POINT('Origin',(0.,0.75,0.));
#22903=CARTESIAN_POINT('',(0.775176467748211,0.75,0.977857337884349));
#22904=CARTESIAN_POINT('Origin',(0.721999869202979,0.75,0.993747566553533));
#22905=CARTESIAN_POINT('',(0.844553975349804,0.75,0.918603348636233));
#22906=CARTESIAN_POINT('Origin',(0.,0.75,0.));
#22907=CARTESIAN_POINT('',(0.918603348636233,0.75,0.844553975349804));
#22908=CARTESIAN_POINT('Origin',(0.86856722168183,0.75,0.86856722168183));
#22909=CARTESIAN_POINT('',(0.977857337884349,0.75,0.775176467748211));
#22910=CARTESIAN_POINT('Origin',(0.,0.75,0.));
#22911=CARTESIAN_POINT('',(1.0394111664111,0.75,0.690454891028201));
#22912=CARTESIAN_POINT('Origin',(0.993747566553533,0.75,0.72199986920298));
#22913=CARTESIAN_POINT('',(1.08708260743774,0.75,0.612662169561029));
#22914=CARTESIAN_POINT('Origin',(0.,0.75,0.));
#22915=CARTESIAN_POINT('',(1.13462523166105,0.75,0.519354515801077));
#22916=CARTESIAN_POINT('Origin',(1.0944585482776,0.75,0.557654483764164));
#22917=CARTESIAN_POINT('',(1.16954029537568,0.75,0.435062095450087));
#22918=CARTESIAN_POINT('Origin',(0.,0.75,0.));
#22919=CARTESIAN_POINT('',(1.20190105810224,0.75,0.335465908756113));
#22920=CARTESIAN_POINT('Origin',(1.1682203282434,0.75,0.379577794185952));
#22921=CARTESIAN_POINT('Origin',(0.,0.75,0.));
#22922=CARTESIAN_POINT('Origin',(0.,0.75,0.));
#22923=CARTESIAN_POINT('',(-1.4,0.85,1.71450551880629E-16));
#22924=CARTESIAN_POINT('Origin',(0.,0.85,0.));
#22925=CARTESIAN_POINT('',(-1.4,0.75,1.71450551880629E-16));
#22926=CARTESIAN_POINT('Origin',(0.,0.85,0.));
#22927=CARTESIAN_POINT('Origin',(1.21321664662686,0.,0.192154639568406));
#22928=CARTESIAN_POINT('',(1.23958209161204,0.,0.14331701769005));
#22929=CARTESIAN_POINT('',(1.22320001975977,0.,0.246749348660855));
#22930=CARTESIAN_POINT('Origin',(0.,0.,0.));
#22931=CARTESIAN_POINT('',(1.20190105810224,0.,0.33546590875611));
#22932=CARTESIAN_POINT('Origin',(1.1682203282434,0.,0.379577794185952));
#22933=CARTESIAN_POINT('',(1.16954029537568,0.,0.43506209545009));
#22934=CARTESIAN_POINT('Origin',(0.,0.,0.));
#22935=CARTESIAN_POINT('',(1.13462523166105,0.,0.519354515801074));
#22936=CARTESIAN_POINT('Origin',(1.0944585482776,0.,0.557654483764164));
#22937=CARTESIAN_POINT('',(1.08708260743774,0.,0.612662169561031));
#22938=CARTESIAN_POINT('Origin',(0.,0.,0.));
#22939=CARTESIAN_POINT('',(1.03941116641111,0.,0.690454891028199));
#22940=CARTESIAN_POINT('Origin',(0.993747566553533,0.,0.72199986920298));
#22941=CARTESIAN_POINT('',(0.977857337884347,0.,0.775176467748214));
#22942=CARTESIAN_POINT('Origin',(0.,0.,0.));
#22943=CARTESIAN_POINT('',(0.918603348636235,0.,0.844553975349802));
#22944=CARTESIAN_POINT('Origin',(0.86856722168183,0.,0.86856722168183));
#22945=CARTESIAN_POINT('',(0.844553975349802,0.,0.918603348636235));
#22946=CARTESIAN_POINT('Origin',(0.,0.,0.));
#22947=CARTESIAN_POINT('',(0.775176467748213,0.,0.977857337884347));
#22948=CARTESIAN_POINT('Origin',(0.721999869202979,0.,0.993747566553533));
#22949=CARTESIAN_POINT('',(0.690454891028198,0.,1.03941116641111));
#22950=CARTESIAN_POINT('Origin',(0.,0.,0.));
#22951=CARTESIAN_POINT('',(0.612662169561031,0.,1.08708260743774));
#22952=CARTESIAN_POINT('Origin',(0.557654483764164,0.,1.0944585482776));
#22953=CARTESIAN_POINT('',(0.519354515801074,0.,1.13462523166105));
#22954=CARTESIAN_POINT('Origin',(0.,0.,0.));
#22955=CARTESIAN_POINT('',(0.43506209545009,0.,1.16954029537568));
#22956=CARTESIAN_POINT('Origin',(0.379577794185951,0.,1.1682203282434));
#22957=CARTESIAN_POINT('',(0.33546590875611,0.,1.20190105810224));
#22958=CARTESIAN_POINT('Origin',(0.,0.,0.));
#22959=CARTESIAN_POINT('',(0.246749348660854,0.,1.22320001975977));
#22960=CARTESIAN_POINT('Origin',(0.192154639568406,0.,1.21321664662686));
#22961=CARTESIAN_POINT('',(0.14331701769005,0.,1.23958209161204));
#22962=CARTESIAN_POINT('Origin',(0.,0.,0.));
#22963=CARTESIAN_POINT('',(0.0523608139934508,0.,1.24674050008925));
#22964=CARTESIAN_POINT('Origin',(-2.25642313758905E-16,0.,1.22833954473516));
#22965=CARTESIAN_POINT('',(-0.0523608139934513,0.,1.24674050008925));
#22966=CARTESIAN_POINT('Origin',(0.,0.,0.));
#22967=CARTESIAN_POINT('',(-0.14331701769005,0.,1.23958209161204));
#22968=CARTESIAN_POINT('Origin',(-0.192154639568406,0.,1.21321664662686));
#22969=CARTESIAN_POINT('',(-0.246749348660855,0.,1.22320001975977));
#22970=CARTESIAN_POINT('Origin',(0.,0.,0.));
#22971=CARTESIAN_POINT('',(-0.33546590875611,0.,1.20190105810224));
#22972=CARTESIAN_POINT('Origin',(-0.379577794185951,0.,1.1682203282434));
#22973=CARTESIAN_POINT('',(-0.43506209545009,0.,1.16954029537568));
#22974=CARTESIAN_POINT('Origin',(0.,0.,0.));
#22975=CARTESIAN_POINT('',(-0.519354515801074,0.,1.13462523166105));
#22976=CARTESIAN_POINT('Origin',(-0.557654483764164,0.,1.0944585482776));
#22977=CARTESIAN_POINT('',(-0.612662169561031,0.,1.08708260743774));
#22978=CARTESIAN_POINT('Origin',(0.,0.,0.));
#22979=CARTESIAN_POINT('',(-0.690454891028199,0.,1.03941116641111));
#22980=CARTESIAN_POINT('Origin',(-0.721999869202979,0.,0.993747566553533));
#22981=CARTESIAN_POINT('',(-0.775176467748213,0.,0.977857337884347));
#22982=CARTESIAN_POINT('Origin',(0.,0.,0.));
#22983=CARTESIAN_POINT('',(-0.844553975349802,0.,0.918603348636235));
#22984=CARTESIAN_POINT('Origin',(-0.86856722168183,0.,0.86856722168183));
#22985=CARTESIAN_POINT('',(-0.918603348636235,0.,0.844553975349802));
#22986=CARTESIAN_POINT('Origin',(0.,0.,0.));
#22987=CARTESIAN_POINT('',(-0.977857337884347,0.,0.775176467748213));
#22988=CARTESIAN_POINT('Origin',(-0.993747566553533,0.,0.721999869202979));
#22989=CARTESIAN_POINT('',(-1.03941116641111,0.,0.690454891028198));
#22990=CARTESIAN_POINT('Origin',(0.,0.,0.));
#22991=CARTESIAN_POINT('',(-1.08708260743774,0.,0.612662169561031));
#22992=CARTESIAN_POINT('Origin',(-1.0944585482776,0.,0.557654483764164));
#22993=CARTESIAN_POINT('',(-1.13462523166105,0.,0.519354515801074));
#22994=CARTESIAN_POINT('Origin',(0.,0.,0.));
#22995=CARTESIAN_POINT('',(-1.16954029537568,0.,0.43506209545009));
#22996=CARTESIAN_POINT('Origin',(-1.1682203282434,0.,0.379577794185951));
#22997=CARTESIAN_POINT('',(-1.20190105810224,0.,0.33546590875611));
#22998=CARTESIAN_POINT('Origin',(0.,0.,0.));
#22999=CARTESIAN_POINT('',(-1.22320001975977,0.,0.246749348660854));
#23000=CARTESIAN_POINT('Origin',(-1.21321664662686,0.,0.192154639568406));
#23001=CARTESIAN_POINT('',(-1.23958209161204,0.,0.14331701769005));
#23002=CARTESIAN_POINT('Origin',(0.,0.,0.));
#23003=CARTESIAN_POINT('',(-1.24674050008925,0.,0.0523608139934509));
#23004=CARTESIAN_POINT('Origin',(-1.22833954473516,0.,-1.50428209172603E-16));
#23005=CARTESIAN_POINT('',(-1.24674050008925,0.,-0.0523608139934512));
#23006=CARTESIAN_POINT('Origin',(0.,0.,0.));
#23007=CARTESIAN_POINT('',(-1.23958209161204,0.,-0.14331701769005));
#23008=CARTESIAN_POINT('Origin',(-1.21321664662686,0.,-0.192154639568406));
#23009=CARTESIAN_POINT('',(-1.22320001975977,0.,-0.246749348660855));
#23010=CARTESIAN_POINT('Origin',(0.,0.,0.));
#23011=CARTESIAN_POINT('',(-1.20190105810224,0.,-0.33546590875611));
#23012=CARTESIAN_POINT('Origin',(-1.1682203282434,0.,-0.379577794185951));
#23013=CARTESIAN_POINT('',(-1.16954029537568,0.,-0.43506209545009));
#23014=CARTESIAN_POINT('Origin',(0.,0.,0.));
#23015=CARTESIAN_POINT('',(-1.13462523166105,0.,-0.519354515801074));
#23016=CARTESIAN_POINT('Origin',(-1.0944585482776,0.,-0.557654483764164));
#23017=CARTESIAN_POINT('',(-1.08708260743774,0.,-0.612662169561031));
#23018=CARTESIAN_POINT('Origin',(0.,0.,0.));
#23019=CARTESIAN_POINT('',(-1.03941116641111,0.,-0.690454891028199));
#23020=CARTESIAN_POINT('Origin',(-0.993747566553533,0.,-0.721999869202979));
#23021=CARTESIAN_POINT('',(-0.977857337884347,0.,-0.775176467748213));
#23022=CARTESIAN_POINT('Origin',(0.,0.,0.));
#23023=CARTESIAN_POINT('',(-0.918603348636235,0.,-0.844553975349802));
#23024=CARTESIAN_POINT('Origin',(-0.86856722168183,0.,-0.86856722168183));
#23025=CARTESIAN_POINT('',(-0.844553975349802,0.,-0.918603348636235));
#23026=CARTESIAN_POINT('Origin',(0.,0.,0.));
#23027=CARTESIAN_POINT('',(-0.775176467748213,0.,-0.977857337884347));
#23028=CARTESIAN_POINT('Origin',(-0.721999869202979,0.,-0.993747566553533));
#23029=CARTESIAN_POINT('',(-0.690454891028198,0.,-1.03941116641111));
#23030=CARTESIAN_POINT('Origin',(0.,0.,0.));
#23031=CARTESIAN_POINT('',(-0.612662169561031,0.,-1.08708260743774));
#23032=CARTESIAN_POINT('Origin',(-0.557654483764164,0.,-1.0944585482776));
#23033=CARTESIAN_POINT('',(-0.519354515801074,0.,-1.13462523166105));
#23034=CARTESIAN_POINT('Origin',(0.,0.,0.));
#23035=CARTESIAN_POINT('',(-0.43506209545009,0.,-1.16954029537568));
#23036=CARTESIAN_POINT('Origin',(-0.379577794185951,0.,-1.1682203282434));
#23037=CARTESIAN_POINT('',(-0.33546590875611,0.,-1.20190105810224));
#23038=CARTESIAN_POINT('Origin',(0.,0.,0.));
#23039=CARTESIAN_POINT('',(-0.246749348660854,0.,-1.22320001975977));
#23040=CARTESIAN_POINT('Origin',(-0.192154639568406,0.,-1.21321664662686));
#23041=CARTESIAN_POINT('',(-0.14331701769005,0.,-1.23958209161204));
#23042=CARTESIAN_POINT('Origin',(0.,0.,0.));
#23043=CARTESIAN_POINT('',(-0.052360813993451,0.,-1.24674050008925));
#23044=CARTESIAN_POINT('Origin',(7.52141045863017E-17,0.,-1.22833954473516));
#23045=CARTESIAN_POINT('',(0.0523608139934511,0.,-1.24674050008925));
#23046=CARTESIAN_POINT('Origin',(0.,0.,0.));
#23047=CARTESIAN_POINT('',(0.14331701769005,0.,-1.23958209161204));
#23048=CARTESIAN_POINT('Origin',(0.192154639568406,0.,-1.21321664662686));
#23049=CARTESIAN_POINT('',(0.246749348660855,0.,-1.22320001975977));
#23050=CARTESIAN_POINT('Origin',(0.,0.,0.));
#23051=CARTESIAN_POINT('',(0.33546590875611,0.,-1.20190105810224));
#23052=CARTESIAN_POINT('Origin',(0.379577794185951,0.,-1.1682203282434));
#23053=CARTESIAN_POINT('',(0.43506209545009,0.,-1.16954029537568));
#23054=CARTESIAN_POINT('Origin',(0.,0.,0.));
#23055=CARTESIAN_POINT('',(0.519354515801074,0.,-1.13462523166105));
#23056=CARTESIAN_POINT('Origin',(0.557654483764164,0.,-1.0944585482776));
#23057=CARTESIAN_POINT('',(0.612662169561031,0.,-1.08708260743774));
#23058=CARTESIAN_POINT('Origin',(0.,0.,0.));
#23059=CARTESIAN_POINT('',(0.690454891028198,0.,-1.03941116641111));
#23060=CARTESIAN_POINT('Origin',(0.721999869202979,0.,-0.993747566553533));
#23061=CARTESIAN_POINT('',(0.775176467748213,0.,-0.977857337884347));
#23062=CARTESIAN_POINT('Origin',(0.,0.,0.));
#23063=CARTESIAN_POINT('',(0.844553975349802,0.,-0.918603348636235));
#23064=CARTESIAN_POINT('Origin',(0.86856722168183,0.,-0.86856722168183));
#23065=CARTESIAN_POINT('',(0.918603348636235,0.,-0.844553975349802));
#23066=CARTESIAN_POINT('Origin',(0.,0.,0.));
#23067=CARTESIAN_POINT('',(0.977857337884347,0.,-0.775176467748213));
#23068=CARTESIAN_POINT('Origin',(0.993747566553533,0.,-0.721999869202979));
#23069=CARTESIAN_POINT('',(1.03941116641111,0.,-0.690454891028198));
#23070=CARTESIAN_POINT('Origin',(0.,0.,0.));
#23071=CARTESIAN_POINT('',(1.08708260743774,0.,-0.612662169561031));
#23072=CARTESIAN_POINT('Origin',(1.0944585482776,0.,-0.557654483764164));
#23073=CARTESIAN_POINT('',(1.13462523166105,0.,-0.519354515801074));
#23074=CARTESIAN_POINT('Origin',(0.,0.,0.));
#23075=CARTESIAN_POINT('',(1.16954029537568,0.,-0.43506209545009));
#23076=CARTESIAN_POINT('Origin',(1.1682203282434,0.,-0.379577794185951));
#23077=CARTESIAN_POINT('',(1.20190105810224,0.,-0.33546590875611));
#23078=CARTESIAN_POINT('Origin',(0.,0.,0.));
#23079=CARTESIAN_POINT('',(1.22320001975977,0.,-0.246749348660855));
#23080=CARTESIAN_POINT('Origin',(1.21321664662686,0.,-0.192154639568406));
#23081=CARTESIAN_POINT('',(1.23958209161204,0.,-0.14331701769005));
#23082=CARTESIAN_POINT('Origin',(0.,0.,0.));
#23083=CARTESIAN_POINT('',(1.24674050008925,0.,0.052360813993451));
#23084=CARTESIAN_POINT('Origin',(1.22833954473516,0.,0.));
#23085=CARTESIAN_POINT('',(1.24674050008925,0.,-0.052360813993451));
#23086=CARTESIAN_POINT('Origin',(0.,0.,0.));
#23516=UNCERTAINTY_MEASURE_WITH_UNIT(LENGTH_MEASURE(0.001),#23588,
'DISTANCE_ACCURACY_VALUE',
'Maximum model space distance between geometric entities at asserted c
onnectivities');
#23522=UNCERTAINTY_MEASURE_WITH_UNIT(LENGTH_MEASURE(0.001),#23588,
'DISTANCE_ACCURACY_VALUE',
'Maximum model space distance between geometric entities at asserted c
onnectivities');
#23581=(
GEOMETRIC_REPRESENTATION_CONTEXT(3)
GLOBAL_UNCERTAINTY_ASSIGNED_CONTEXT((#23516))
GLOBAL_UNIT_ASSIGNED_CONTEXT((#23588,#23590,#23591))
REPRESENTATION_CONTEXT('','3D')
);
#23587=(
GEOMETRIC_REPRESENTATION_CONTEXT(3)
GLOBAL_UNCERTAINTY_ASSIGNED_CONTEXT((#23522))
GLOBAL_UNIT_ASSIGNED_CONTEXT((#23588,#23590,#23591))
REPRESENTATION_CONTEXT('','3D')
);
#23588=(
LENGTH_UNIT()
NAMED_UNIT(*)
SI_UNIT(.CENTI.,.METRE.)
);
#23590=(
NAMED_UNIT(*)
PLANE_ANGLE_UNIT()
SI_UNIT($,.RADIAN.)
);
#23591=(
NAMED_UNIT(*)
SI_UNIT($,.STERADIAN.)
SOLID_ANGLE_UNIT()
);
#23650=SHAPE_DEFINITION_REPRESENTATION(#23727,#23883);
#23727=PRODUCT_DEFINITION_SHAPE('',$,#23948);
#23883=SHAPE_REPRESENTATION('',(#14071),#23581);
#23889=PRODUCT_DEFINITION_CONTEXT('part definition',#24083,'design');
#23948=PRODUCT_DEFINITION(
'Timing Pulley - 2 mm Pitch, 40 Teeth, 12 mm Bore',
'Timing Pulley - 2 mm Pitch, 40 Teeth, 12 mm Bore',#24012,#23889);
#24012=PRODUCT_DEFINITION_FORMATION('',$,#24143);
#24083=APPLICATION_CONTEXT(
'Core Data for Automotive Mechanical Design Process');
#24084=PRODUCT_CONTEXT('part definition',#24083,'mechanical');
#24143=PRODUCT('Timing Pulley - 2 mm Pitch, 40 Teeth, 12 mm Bore',
'Timing Pulley - 2 mm Pitch, 40 Teeth, 12 mm Bore',
'Timing Pulley - 2 mm Pitch, 40 Teeth, 12 mm Bore',(#24084));
#24198=COLOUR_RGB('Sky Blue',0.24,0.69,0.87);
#24199=FILL_AREA_STYLE_COLOUR('',#24198);
#24200=FILL_AREA_STYLE('',(#24199));
#24201=SURFACE_STYLE_FILL_AREA(#24200);
#24202=SURFACE_SIDE_STYLE('',(#24201));
#24203=SURFACE_STYLE_USAGE(.BOTH.,#24202);
#24204=PRESENTATION_STYLE_ASSIGNMENT((#24203));
ENDSEC;
END-ISO-10303-21;
